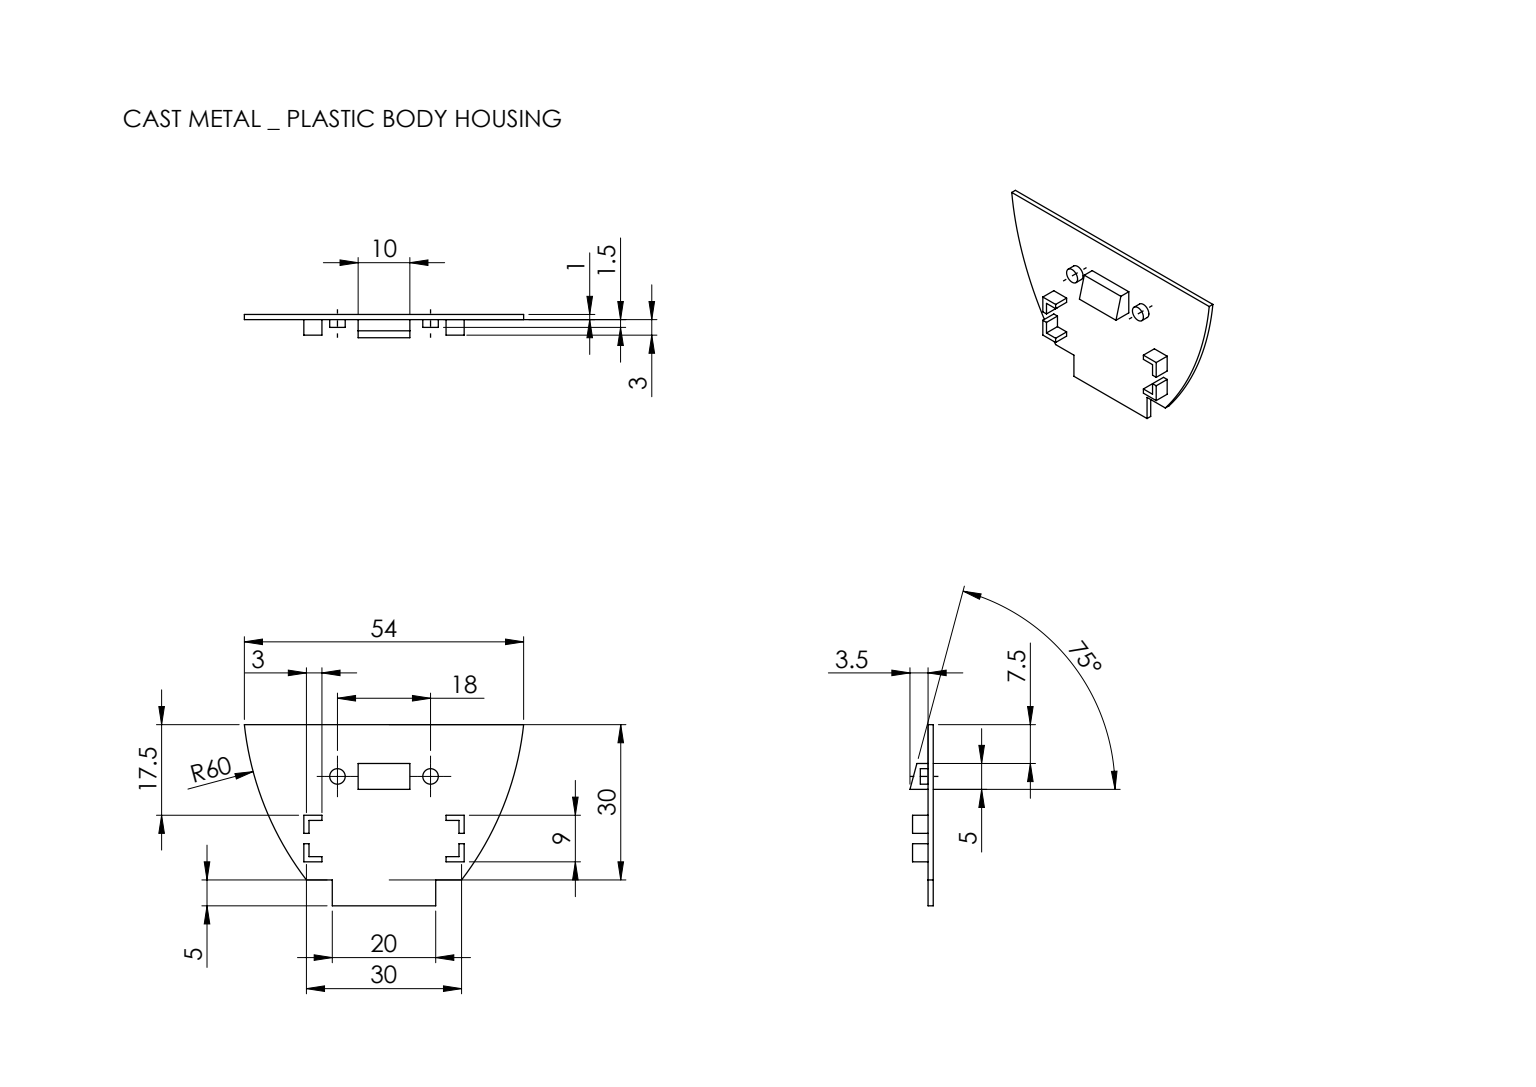
ISO-10303-21;
HEADER;
FILE_DESCRIPTION (('STEP AP214'),
    '1' );
FILE_NAME ('Cast Metal _ Plastic Body Housing.step',
    '2026-10-04T16:38:04',
    ( '' ),
    ( '' ),
    'SwSTEP 2.0',
    'SolidWorks 2026',
    '' );
FILE_SCHEMA (( 'AUTOMOTIVE_DESIGN' ));
ENDSEC;

DATA;
#46=DIRECTION ( 'NONE',  ( 1.000000000000000000, -6.938893903907222067E-15, 0.000000000000000000 ) ) ;
#48=EDGE_LOOP ( 'NONE', ( #6607, #18673, #6407, #16806 ) ) ;
#59=LINE ( 'NONE', #8216, #18452 ) ;
#71=ORIENTED_EDGE ( 'NONE', *, *, #17925, .T. ) ;
#150=EDGE_CURVE ( 'NONE', #20096, #3927, #16331, .T. ) ;
#155=EDGE_CURVE ( 'NONE', #9432, #10023, #14985, .T. ) ;
#189=ORIENTED_EDGE ( 'NONE', *, *, #9219, .F. ) ;
#198=EDGE_LOOP ( 'NONE', ( #19605, #1454, #13205, #13918 ) ) ;
#200=VERTEX_POINT ( 'NONE', #10184 ) ;
#212=DIRECTION ( 'NONE',  ( -1.000000000000000000, -6.938893903907222067E-15, 0.000000000000000000 ) ) ;
#216=ORIENTED_EDGE ( 'NONE', *, *, #5288, .T. ) ;
#237=CARTESIAN_POINT ( 'NONE',  ( 11.99999999999999822, -25.50000000000000355, 4.000000000000000000 ) ) ;
#244=ORIENTED_EDGE ( 'NONE', *, *, #20430, .T. ) ;
#247=LINE ( 'NONE', #19711, #19278 ) ;
#253=DIRECTION ( 'NONE',  ( 0.000000000000000000, 0.000000000000000000, -1.000000000000000000 ) ) ;
#254=EDGE_CURVE ( 'NONE', #12726, #11061, #10084, .T. ) ;
#255=CARTESIAN_POINT ( 'NONE',  ( -15.49999999999998046, -26.49999999999999645, 4.000000000000000000 ) ) ;
#297=VECTOR ( 'NONE', #5292, 1000.000000000000000 ) ;
#329=ORIENTED_EDGE ( 'NONE', *, *, #3787, .F. ) ;
#382=VERTEX_POINT ( 'NONE', #11949 ) ;
#383=ADVANCED_FACE ( 'NONE', ( #12259 ), #18550, .T. ) ;
#386=CARTESIAN_POINT ( 'NONE',  ( -14.99999999999998046, -26.49999999999999645, 4.000000000000000000 ) ) ;
#387=VECTOR ( 'NONE', #11320, 1000.000000000000000 ) ;
#398=AXIS2_PLACEMENT_3D ( 'NONE', #19475, #19368, #6705 ) ;
#408=ORIENTED_EDGE ( 'NONE', *, *, #19426, .T. ) ;
#437=DIRECTION ( 'NONE',  ( 1.000000000000000000, 5.204170427930411817E-15, -0.000000000000000000 ) ) ;
#452=VECTOR ( 'NONE', #1980, 1000.000000000000000 ) ;
#459=ADVANCED_FACE ( 'NONE', ( #3832 ), #17953, .T. ) ;
#462=DIRECTION ( 'NONE',  ( 1.000000000000000000, 0.000000000000000000, -0.000000000000000000 ) ) ;
#486=CARTESIAN_POINT ( 'NONE',  ( 15.00000000000001776, -26.49999999999999645, 1.000000000000000000 ) ) ;
#491=PLANE ( 'NONE',  #4290 ) ;
#498=ORIENTED_EDGE ( 'NONE', *, *, #11572, .F. ) ;
#514=VECTOR ( 'NONE', #18897, 1000.000000000000000 ) ;
#520=EDGE_CURVE ( 'NONE', #9432, #6659, #2464, .T. ) ;
#522=PLANE ( 'NONE',  #398 ) ;
#523=VECTOR ( 'NONE', #704, 1000.000000000000000 ) ;
#526=ORIENTED_EDGE ( 'NONE', *, *, #18607, .T. ) ;
#530=ADVANCED_FACE ( 'NONE', ( #697 ), #13548, .T. ) ;
#533=DIRECTION ( 'NONE',  ( 0.000000000000000000, 0.000000000000000000, 1.000000000000000000 ) ) ;
#535=FACE_OUTER_BOUND ( 'NONE', #13184, .T. ) ;
#551=VERTEX_POINT ( 'NONE', #2158 ) ;
#568=CARTESIAN_POINT ( 'NONE',  ( 15.50000000000000178, -20.99999999999999645, 4.000000000000000000 ) ) ;
#579=ORIENTED_EDGE ( 'NONE', *, *, #13507, .T. ) ;
#581=CARTESIAN_POINT ( 'NONE',  ( 15.50000000000000178, -23.00000000000000711, 1.000000000000000000 ) ) ;
#585=EDGE_LOOP ( 'NONE', ( #6013, #20660, #8946, #16986 ) ) ;
#599=EDGE_LOOP ( 'NONE', ( #16407, #1610, #13461, #14948 ) ) ;
#603=DIRECTION ( 'NONE',  ( 5.204170427930411817E-15, -1.000000000000000000, 0.000000000000000000 ) ) ;
#628=VECTOR ( 'NONE', #3098, 1000.000000000000000 ) ;
#642=VECTOR ( 'NONE', #3133, 1000.000000000000000 ) ;
#668=VECTOR ( 'NONE', #922, 1000.000000000000000 ) ;
#688=EDGE_LOOP ( 'NONE', ( #8301, #4160, #16182, #17775 ) ) ;
#697=FACE_OUTER_BOUND ( 'NONE', #48, .T. ) ;
#704=DIRECTION ( 'NONE',  ( -0.000000000000000000, -0.000000000000000000, -1.000000000000000000 ) ) ;
#722=CARTESIAN_POINT ( 'NONE',  ( 4.000000000000000000, -12.50000000000000000, 1.000000000000000000 ) ) ;
#745=AXIS2_PLACEMENT_3D ( 'NONE', #893, #13543, #3828 ) ;
#754=PRESENTATION_STYLE_ASSIGNMENT (( #11425 ) ) ;
#757=VECTOR ( 'NONE', #16963, 1000.000000000000000 ) ;
#787=ORIENTED_EDGE ( 'NONE', *, *, #12469, .F. ) ;
#794=LINE ( 'NONE', #11664, #1088 ) ;
#817=EDGE_LOOP ( 'NONE', ( #11943, #5676, #6063, #12462 ) ) ;
#831=ADVANCED_FACE ( 'NONE', ( #10843 ), #17206, .F. ) ;
#844=FILL_AREA_STYLE ('',( #8584 ) ) ;
#846=LINE ( 'NONE', #4289, #16135 ) ;
#849=CARTESIAN_POINT ( 'NONE',  ( -9.000000000000000000, -9.999999999999992895, 2.500000000000000000 ) ) ;
#868=VERTEX_POINT ( 'NONE', #2989 ) ;
#872=CARTESIAN_POINT ( 'NONE',  ( -27.00000000000000000, 0.000000000000000000, 1.000000000000000000 ) ) ;
#877=CARTESIAN_POINT ( 'NONE',  ( -12.00000000000000000, -25.49999999999998934, 4.000000000000000000 ) ) ;
#881=ORIENTED_EDGE ( 'NONE', *, *, #13059, .T. ) ;
#890=ORIENTED_EDGE ( 'NONE', *, *, #18715, .T. ) ;
#893=CARTESIAN_POINT ( 'NONE',  ( 32.65117217603048516, 6.460468870412194420, 0.000000000000000000 ) ) ;
#902=LINE ( 'NONE', #13241, #9957 ) ;
#911=VERTEX_POINT ( 'NONE', #11044 ) ;
#917=ORIENTED_EDGE ( 'NONE', *, *, #11391, .F. ) ;
#922=DIRECTION ( 'NONE',  ( -0.000000000000000000, -0.000000000000000000, -1.000000000000000000 ) ) ;
#967=FACE_OUTER_BOUND ( 'NONE', #17994, .T. ) ;
#990=AXIS2_PLACEMENT_3D ( 'NONE', #20222, #5883, #4722 ) ;
#1027=ORIENTED_EDGE ( 'NONE', *, *, #17853, .T. ) ;
#1035=PLANE ( 'NONE',  #7985 ) ;
#1036=FACE_OUTER_BOUND ( 'NONE', #17096, .T. ) ;
#1044=ORIENTED_EDGE ( 'NONE', *, *, #9355, .F. ) ;
#1057=ORIENTED_EDGE ( 'NONE', *, *, #3262, .T. ) ;
#1088=VECTOR ( 'NONE', #11873, 1000.000000000000000 ) ;
#1110=EDGE_CURVE ( 'NONE', #4929, #14114, #16258, .T. ) ;
#1124=PLANE ( 'NONE',  #12366 ) ;
#1151=CARTESIAN_POINT ( 'NONE',  ( -9.999999999999998224, -30.00000000000000355, 1.000000000000000000 ) ) ;
#1155=ORIENTED_EDGE ( 'NONE', *, *, #14762, .T. ) ;
#1195=EDGE_CURVE ( 'NONE', #18185, #20045, #9975, .T. ) ;
#1199=LINE ( 'NONE', #4441, #1374 ) ;
#1219=DIRECTION ( 'NONE',  ( -1.000000000000000000, 2.312964634635752916E-15, 0.000000000000000000 ) ) ;
#1231=VERTEX_POINT ( 'NONE', #2334 ) ;
#1244=CARTESIAN_POINT ( 'NONE',  ( 5.000000000000000000, -12.50000000000000000, 4.500000000000000888 ) ) ;
#1245=AXIS2_PLACEMENT_3D ( 'NONE', #6195, #6294, #8185 ) ;
#1255=DIRECTION ( 'NONE',  ( -3.469446951953611033E-15, -1.000000000000000000, 0.000000000000000000 ) ) ;
#1266=FACE_OUTER_BOUND ( 'NONE', #2611, .T. ) ;
#1276=ORIENTED_EDGE ( 'NONE', *, *, #16635, .F. ) ;
#1282=UNCERTAINTY_MEASURE_WITH_UNIT (LENGTH_MEASURE( 1.000000000000000082E-05 ), #8702, 'distance_accuracy_value', 'NONE');
#1284=DIRECTION ( 'NONE',  ( 3.469446951953611033E-15, 1.000000000000000000, 0.000000000000000000 ) ) ;
#1358=VECTOR ( 'NONE', #18316, 1000.000000000000000 ) ;
#1367=CARTESIAN_POINT ( 'NONE',  ( 15.00000000000001421, -29.99999999999998579, 0.000000000000000000 ) ) ;
#1374=VECTOR ( 'NONE', #12173, 1000.000000000000000 ) ;
#1375=VECTOR ( 'NONE', #5558, 1000.000000000000000 ) ;
#1408=EDGE_LOOP ( 'NONE', ( #15317, #16815, #12977, #18861, #4503, #15029 ) ) ;
#1412=DIRECTION ( 'NONE',  ( -6.938893903907222067E-15, -1.000000000000000000, 0.000000000000000000 ) ) ;
#1414=ORIENTED_EDGE ( 'NONE', *, *, #6972, .T. ) ;
#1424=CARTESIAN_POINT ( 'NONE',  ( -27.00000000000000000, 0.000000000000000000, 0.000000000000000000 ) ) ;
#1432=VECTOR ( 'NONE', #9969, 1000.000000000000000 ) ;
#1434=VERTEX_POINT ( 'NONE', #18655 ) ;
#1435=EDGE_CURVE ( 'NONE', #7660, #4902, #17180, .T. ) ;
#1454=ORIENTED_EDGE ( 'NONE', *, *, #17925, .F. ) ;
#1460=FACE_OUTER_BOUND ( 'NONE', #585, .T. ) ;
#1482=ORIENTED_EDGE ( 'NONE', *, *, #16635, .T. ) ;
#1489=CARTESIAN_POINT ( 'NONE',  ( -11.99999999999999467, -17.50000000000000000, 1.000000000000000000 ) ) ;
#1516=FACE_BOUND ( 'NONE', #16320, .T. ) ;
#1549=ORIENTED_EDGE ( 'NONE', *, *, #1825, .F. ) ;
#1557=ORIENTED_EDGE ( 'NONE', *, *, #15424, .F. ) ;
#1562=LINE ( 'NONE', #3235, #13129 ) ;
#1565=CARTESIAN_POINT ( 'NONE',  ( 4.000000000000000000, 0.000000000000000000, 0.000000000000000000 ) ) ;
#1571=PLANE ( 'NONE',  #11672 ) ;
#1594=LINE ( 'NONE', #7781, #15066 ) ;
#1601=VECTOR ( 'NONE', #13561, 1000.000000000000000 ) ;
#1604=ORIENTED_EDGE ( 'NONE', *, *, #18607, .F. ) ;
#1607=PLANE ( 'NONE',  #6334 ) ;
#1610=ORIENTED_EDGE ( 'NONE', *, *, #11754, .F. ) ;
#1620=DIRECTION ( 'NONE',  ( -1.000000000000000000, -3.469446951953611033E-15, 0.000000000000000000 ) ) ;
#1632=VECTOR ( 'NONE', #7369, 1000.000000000000000 ) ;
#1642=CARTESIAN_POINT ( 'NONE',  ( 10.00000000000000533, -30.00000000000000355, 0.000000000000000000 ) ) ;
#1647=LINE ( 'NONE', #12619, #3950 ) ;
#1695=ORIENTED_EDGE ( 'NONE', *, *, #9410, .F. ) ;
#1776=DIRECTION ( 'NONE',  ( -1.000000000000000000, 0.000000000000000000, 0.000000000000000000 ) ) ;
#1777=DIRECTION ( 'NONE',  ( 0.000000000000000000, -0.9659258262890672020, 0.2588190451025245142 ) ) ;
#1793=CARTESIAN_POINT ( 'NONE',  ( 0.000000000000000000, 0.000000000000000000, 0.000000000000000000 ) ) ;
#1799=PLANE ( 'NONE',  #15935 ) ;
#1820=ORIENTED_EDGE ( 'NONE', *, *, #15526, .F. ) ;
#1825=EDGE_CURVE ( 'NONE', #8456, #2576, #5382, .T. ) ;
#1828=CARTESIAN_POINT ( 'NONE',  ( 12.00000000000000178, -26.50000000000000355, 4.000000000000000000 ) ) ;
#1832=CARTESIAN_POINT ( 'NONE',  ( 15.00000000000001421, -25.49999999999999645, 1.000000000000000000 ) ) ;
#1845=ORIENTED_EDGE ( 'NONE', *, *, #9443, .T. ) ;
#1846=DIRECTION ( 'NONE',  ( 0.000000000000000000, -0.9659258262890672020, 0.2588190451025246253 ) ) ;
#1866=VERTEX_POINT ( 'NONE', #5666 ) ;
#1869=EDGE_LOOP ( 'NONE', ( #11250, #11872, #14832, #4061 ) ) ;
#1886=EDGE_CURVE ( 'NONE', #200, #2500, #20000, .T. ) ;
#1893=ORIENTED_EDGE ( 'NONE', *, *, #3662, .F. ) ;
#1900=LINE ( 'NONE', #11214, #20633 ) ;
#1901=DIRECTION ( 'NONE',  ( 0.000000000000000000, 0.000000000000000000, 1.000000000000000000 ) ) ;
#1924=CARTESIAN_POINT ( 'NONE',  ( -15.49999999999999822, -20.99999999999999645, 4.000000000000000000 ) ) ;
#1942=VERTEX_POINT ( 'NONE', #10685 ) ;
#1947=DIRECTION ( 'NONE',  ( 1.000000000000000000, 0.000000000000000000, 0.000000000000000000 ) ) ;
#1951=ORIENTED_EDGE ( 'NONE', *, *, #5701, .T. ) ;
#1953=DIRECTION ( 'NONE',  ( 0.000000000000000000, 0.000000000000000000, 1.000000000000000000 ) ) ;
#1978=CARTESIAN_POINT ( 'NONE',  ( -5.000000000000000000, -7.500000000000000000, 3.160254037844365094 ) ) ;
#1980=DIRECTION ( 'NONE',  ( 0.000000000000000000, 0.000000000000000000, -1.000000000000000000 ) ) ;
#1989=AXIS2_PLACEMENT_3D ( 'NONE', #16860, #18234, #9127 ) ;
#1990=EDGE_CURVE ( 'NONE', #13564, #6014, #16746, .T. ) ;
#1995=EDGE_LOOP ( 'NONE', ( #14834, #2151, #15596, #189, #1557, #14199, #4129, #1695 ) ) ;
#2006=PRODUCT_DEFINITION_SHAPE ( 'NONE', 'NONE',  #20327 ) ;
#2030=DIRECTION ( 'NONE',  ( 4.625929269271477434E-15, 1.000000000000000000, 0.000000000000000000 ) ) ;
#2033=CARTESIAN_POINT ( 'NONE',  ( -11.99999999999999467, -17.50000000000000000, 1.000000000000000000 ) ) ;
#2056=LINE ( 'NONE', #2458, #2757 ) ;
#2100=ORIENTED_EDGE ( 'NONE', *, *, #7749, .T. ) ;
#2104=DIRECTION ( 'NONE',  ( 0.000000000000000000, -0.9659258262890672020, 0.2588190451025245142 ) ) ;
#2108=ADVANCED_FACE ( 'NONE', ( #17469 ), #1571, .F. ) ;
#2121=VECTOR ( 'NONE', #12009, 1000.000000000000000 ) ;
#2150=ORIENTED_EDGE ( 'NONE', *, *, #4677, .T. ) ;
#2151=ORIENTED_EDGE ( 'NONE', *, *, #18217, .T. ) ;
#2158=CARTESIAN_POINT ( 'NONE',  ( 4.000000000000000000, -12.50000000000000000, 3.464723819589916154 ) ) ;
#2160=DIRECTION ( 'NONE',  ( -1.000000000000000000, -3.469446951953611033E-15, 0.000000000000000000 ) ) ;
#2167=ORIENTED_EDGE ( 'NONE', *, *, #14644, .T. ) ;
#2195=CARTESIAN_POINT ( 'NONE',  ( 12.00000000000000178, -18.50000000000000355, 1.000000000000000000 ) ) ;
#2200=( LENGTH_UNIT ( ) NAMED_UNIT ( * ) SI_UNIT ( .MILLI., .METRE. ) );
#2202=CARTESIAN_POINT ( 'NONE',  ( -14.49999999999999645, -22.99999999999998579, 4.000000000000000000 ) ) ;
#2228=DIRECTION ( 'NONE',  ( 0.000000000000000000, -1.000000000000000000, 0.000000000000000000 ) ) ;
#2235=LINE ( 'NONE', #6754, #14984 ) ;
#2238=ORIENTED_EDGE ( 'NONE', *, *, #3662, .T. ) ;
#2310=AXIS2_PLACEMENT_3D ( 'NONE', #2824, #11084, #17041 ) ;
#2334=CARTESIAN_POINT ( 'NONE',  ( 5.000000000000000000, -7.500000000000000000, 3.160254037844365094 ) ) ;
#2337=DIRECTION ( 'NONE',  ( -1.000000000000000000, 6.938893903907222067E-15, 0.000000000000000000 ) ) ;
#2353=ORIENTED_EDGE ( 'NONE', *, *, #254, .F. ) ;
#2355=ORIENTED_EDGE ( 'NONE', *, *, #20532, .T. ) ;
#2359=LINE ( 'NONE', #5401, #7994 ) ;
#2378=ORIENTED_EDGE ( 'NONE', *, *, #19426, .F. ) ;
#2383=ORIENTED_EDGE ( 'NONE', *, *, #1435, .T. ) ;
#2390=CARTESIAN_POINT ( 'NONE',  ( 10.49999999999999467, -9.999999999999991118, 2.500000000000000000 ) ) ;
#2455=CARTESIAN_POINT ( 'NONE',  ( 15.50000000000002132, -26.49999999999999645, 1.000000000000000000 ) ) ;
#2458=CARTESIAN_POINT ( 'NONE',  ( 12.00000000000000178, -26.50000000000000355, 1.000000000000000000 ) ) ;
#2464=LINE ( 'NONE', #4042, #297 ) ;
#2467=EDGE_CURVE ( 'NONE', #19883, #3190, #5533, .T. ) ;
#2469=CARTESIAN_POINT ( 'NONE',  ( 5.000000000000000000, -12.50000000000000000, 1.000000000000000000 ) ) ;
#2474=ORIENTED_EDGE ( 'NONE', *, *, #4002, .T. ) ;
#2477=VERTEX_POINT ( 'NONE', #18608 ) ;
#2483=VERTEX_POINT ( 'NONE', #12219 ) ;
#2500=VERTEX_POINT ( 'NONE', #17028 ) ;
#2501=EDGE_CURVE ( 'NONE', #6659, #14414, #4070, .T. ) ;
#2506=( NAMED_UNIT ( * ) SI_UNIT ( $, .STERADIAN. ) SOLID_ANGLE_UNIT ( ) );
#2566=DIRECTION ( 'NONE',  ( 0.000000000000000000, 0.000000000000000000, 1.000000000000000000 ) ) ;
#2576=VERTEX_POINT ( 'NONE', #15251 ) ;
#2600=ORIENTED_EDGE ( 'NONE', *, *, #7451, .T. ) ;
#2611=EDGE_LOOP ( 'NONE', ( #2600, #7746, #1044, #15474 ) ) ;
#2614=ORIENTED_EDGE ( 'NONE', *, *, #1886, .T. ) ;
#2617=LINE ( 'NONE', #15380, #14540 ) ;
#2664=EDGE_LOOP ( 'NONE', ( #6791, #7977 ) ) ;
#2671=VECTOR ( 'NONE', #17590, 1000.000000000000000 ) ;
#2714=ORIENTED_EDGE ( 'NONE', *, *, #11572, .T. ) ;
#2719=LINE ( 'NONE', #10978, #19024 ) ;
#2752=CARTESIAN_POINT ( 'NONE',  ( 10.00000000000000533, -30.00000000000000355, 1.000000000000000000 ) ) ;
#2757=VECTOR ( 'NONE', #5396, 1000.000000000000000 ) ;
#2761=DIRECTION ( 'NONE',  ( -1.000000000000000000, 0.000000000000000000, 0.000000000000000000 ) ) ;
#2767=CARTESIAN_POINT ( 'NONE',  ( -7.500000000000000888, -9.999999999999992895, 1.000000000000000000 ) ) ;
#2777=EDGE_CURVE ( 'NONE', #18339, #6572, #8684, .T. ) ;
#2810=DIRECTION ( 'NONE',  ( 0.000000000000000000, 0.000000000000000000, -1.000000000000000000 ) ) ;
#2813=DIRECTION ( 'NONE',  ( 1.000000000000000000, 0.000000000000000000, 0.000000000000000000 ) ) ;
#2824=CARTESIAN_POINT ( 'NONE',  ( -12.00000000000000000, -25.49999999999998934, 4.000000000000000000 ) ) ;
#2828=PRODUCT ( 'Cast Metal _ Plastic Body Housing', 'Cast Metal _ Plastic Body Housing', '', ( #13255 ) ) ;
#2832=EDGE_LOOP ( 'NONE', ( #2167, #408, #579, #12559, #3746, #13946, #2355, #2238 ) ) ;
#2878=EDGE_CURVE ( 'NONE', #17965, #11811, #14580, .T. ) ;
#2889=FACE_OUTER_BOUND ( 'NONE', #9746, .T. ) ;
#2906=ORIENTED_EDGE ( 'NONE', *, *, #11391, .T. ) ;
#2909=VECTOR ( 'NONE', #5961, 1000.000000000000000 ) ;
#2911=CARTESIAN_POINT ( 'NONE',  ( 27.00000000000000000, 0.000000000000000000, 0.000000000000000000 ) ) ;
#2923=CARTESIAN_POINT ( 'NONE',  ( -14.99999999999998401, -25.49999999999999645, 4.000000000000000000 ) ) ;
#2956=AXIS2_PLACEMENT_3D ( 'NONE', #8491, #18002, #5454 ) ;
#2974=CARTESIAN_POINT ( 'NONE',  ( -11.99999999999999645, -26.49999999999998934, 4.000000000000000000 ) ) ;
#2976=ORIENTED_EDGE ( 'NONE', *, *, #20430, .F. ) ;
#2986=DIRECTION ( 'NONE',  ( -1.000000000000000000, -0.000000000000000000, -0.000000000000000000 ) ) ;
#2989=CARTESIAN_POINT ( 'NONE',  ( -12.00000000000000000, -25.49999999999998934, 4.000000000000000000 ) ) ;
#2999=EDGE_CURVE ( 'NONE', #868, #11896, #3164, .T. ) ;
#3007=ORIENTED_EDGE ( 'NONE', *, *, #5387, .F. ) ;
#3019=CARTESIAN_POINT ( 'NONE',  ( 14.50000000000000000, -23.00000000000001421, 1.000000000000000000 ) ) ;
#3020=CARTESIAN_POINT ( 'NONE',  ( 14.50000000000000000, -20.99999999999998934, 4.000000000000000000 ) ) ;
#3046=VECTOR ( 'NONE', #4131, 1000.000000000000000 ) ;
#3067=CARTESIAN_POINT ( 'NONE',  ( 12.00000000000000178, -26.50000000000000355, 4.000000000000000000 ) ) ;
#3089=VECTOR ( 'NONE', #8023, 1000.000000000000000 ) ;
#3093=CARTESIAN_POINT ( 'NONE',  ( -15.49999999999999822, -22.99999999999999289, 4.000000000000000000 ) ) ;
#3098=DIRECTION ( 'NONE',  ( -1.000000000000000000, -0.000000000000000000, -0.000000000000000000 ) ) ;
#3111=CARTESIAN_POINT ( 'NONE',  ( 15.50000000000000178, -20.99999999999999645, 4.000000000000000000 ) ) ;
#3113=CARTESIAN_POINT ( 'NONE',  ( 15.50000000000000178, -23.00000000000000711, 4.000000000000000000 ) ) ;
#3118=AXIS2_PLACEMENT_3D ( 'NONE', #17355, #11282, #17665 ) ;
#3122=CARTESIAN_POINT ( 'NONE',  ( -4.000000000000000000, -12.50000000000000000, 3.464723819589916154 ) ) ;
#3133=DIRECTION ( 'NONE',  ( 1.000000000000000000, 6.938893903907232322E-16, 0.000000000000000000 ) ) ;
#3144=CARTESIAN_POINT ( 'NONE',  ( -4.000000000000000000, -8.500000000000000000, 2.392927049865408495 ) ) ;
#3164=LINE ( 'NONE', #6409, #13702 ) ;
#3183=CARTESIAN_POINT ( 'NONE',  ( -10.49999999999999822, -9.999999999999992895, 1.000000000000000000 ) ) ;
#3185=ORIENTED_EDGE ( 'NONE', *, *, #1435, .F. ) ;
#3188=EDGE_CURVE ( 'NONE', #16474, #4026, #16739, .T. ) ;
#3190=VERTEX_POINT ( 'NONE', #13496 ) ;
#3191=LINE ( 'NONE', #17904, #16020 ) ;
#3196=CARTESIAN_POINT ( 'NONE',  ( 10.49999999999999645, -9.999999999999991118, 1.000000000000000000 ) ) ;
#3235=CARTESIAN_POINT ( 'NONE',  ( 12.00000000000000178, -18.50000000000000355, 1.000000000000000000 ) ) ;
#3236=ORIENTED_EDGE ( 'NONE', *, *, #13283, .F. ) ;
#3262=EDGE_CURVE ( 'NONE', #12726, #19461, #13391, .T. ) ;
#3307=VECTOR ( 'NONE', #19013, 1000.000000000000000 ) ;
#3311=DIRECTION ( 'NONE',  ( 0.000000000000000000, 0.000000000000000000, -1.000000000000000000 ) ) ;
#3363=EDGE_LOOP ( 'NONE', ( #17972, #9302, #11307, #5959 ) ) ;
#3364=DIRECTION ( 'NONE',  ( 0.000000000000000000, -0.2588190451025247363, -0.9659258262890673130 ) ) ;
#3379=ORIENTED_EDGE ( 'NONE', *, *, #14251, .F. ) ;
#3399=FACE_OUTER_BOUND ( 'NONE', #19377, .T. ) ;
#3407=EDGE_CURVE ( 'NONE', #19990, #7441, #12504, .T. ) ;
#3412=CARTESIAN_POINT ( 'NONE',  ( -10.49999999999999822, -9.999999999999992895, 2.500000000000000000 ) ) ;
#3421=VECTOR ( 'NONE', #18309, 1000.000000000000000 ) ;
#3423=ADVANCED_FACE ( 'NONE', ( #2889 ), #1124, .F. ) ;
#3424=PLANE ( 'NONE',  #8675 ) ;
#3449=ADVANCED_FACE ( 'NONE', ( #18901 ), #4559, .T. ) ;
#3465=EDGE_LOOP ( 'NONE', ( #16160, #5425, #10306, #917, #71, #16273, #4474, #10670 ) ) ;
#3471=FACE_BOUND ( 'NONE', #1995, .T. ) ;
#3505=ORIENTED_EDGE ( 'NONE', *, *, #1195, .T. ) ;
#3509=ORIENTED_EDGE ( 'NONE', *, *, #5846, .T. ) ;
#3539=CARTESIAN_POINT ( 'NONE',  ( 7.500000000000002665, -9.999999999999991118, 2.500000000000000000 ) ) ;
#3547=CARTESIAN_POINT ( 'NONE',  ( 14.50000000000000000, -23.00000000000001421, 4.000000000000000000 ) ) ;
#3548=DIRECTION ( 'NONE',  ( 1.000000000000000000, 2.312964634635756072E-15, 0.000000000000000000 ) ) ;
#3555=FACE_OUTER_BOUND ( 'NONE', #4637, .T. ) ;
#3566=CARTESIAN_POINT ( 'NONE',  ( -14.49999999999998401, -25.49999999999999645, 1.000000000000000000 ) ) ;
#3575=CARTESIAN_POINT ( 'NONE',  ( 27.00000000000000000, 0.000000000000000000, 1.000000000000000000 ) ) ;
#3599=CIRCLE ( 'NONE', #16625, 1.499999999999996225 ) ;
#3611=ORIENTED_EDGE ( 'NONE', *, *, #19595, .F. ) ;
#3644=ORIENTED_EDGE ( 'NONE', *, *, #9219, .T. ) ;
#3662=EDGE_CURVE ( 'NONE', #20379, #13564, #9476, .T. ) ;
#3728=EDGE_LOOP ( 'NONE', ( #17200, #16705, #11798, #9456 ) ) ;
#3733=CARTESIAN_POINT ( 'NONE',  ( 12.00000000000000178, -18.50000000000000355, 4.000000000000000000 ) ) ;
#3746=ORIENTED_EDGE ( 'NONE', *, *, #6940, .T. ) ;
#3776=CARTESIAN_POINT ( 'NONE',  ( 5.000000000000000000, -12.50000000000000000, 1.000000000000000000 ) ) ;
#3779=DIRECTION ( 'NONE',  ( 1.000000000000000000, 2.312964634635756072E-15, 0.000000000000000000 ) ) ;
#3787=EDGE_CURVE ( 'NONE', #17877, #19250, #1199, .T. ) ;
#3828=DIRECTION ( 'NONE',  ( 1.000000000000000000, 0.000000000000000000, 0.000000000000000000 ) ) ;
#3832=FACE_OUTER_BOUND ( 'NONE', #3363, .T. ) ;
#3836=DIRECTION ( 'NONE',  ( -0.000000000000000000, -0.000000000000000000, -1.000000000000000000 ) ) ;
#3874=PRESENTATION_STYLE_ASSIGNMENT (( #16839 ) ) ;
#3894=ORIENTED_EDGE ( 'NONE', *, *, #3407, .F. ) ;
#3922=VERTEX_POINT ( 'NONE', #17089 ) ;
#3923=ORIENTED_EDGE ( 'NONE', *, *, #8620, .F. ) ;
#3927=VERTEX_POINT ( 'NONE', #2767 ) ;
#3941=VERTEX_POINT ( 'NONE', #17396 ) ;
#3950=VECTOR ( 'NONE', #17641, 1000.000000000000000 ) ;
#3955=FACE_OUTER_BOUND ( 'NONE', #9914, .T. ) ;
#3963=ORIENTED_EDGE ( 'NONE', *, *, #150, .T. ) ;
#3972=ORIENTED_EDGE ( 'NONE', *, *, #6354, .F. ) ;
#4002=EDGE_CURVE ( 'NONE', #4902, #3922, #16147, .T. ) ;
#4008=VECTOR ( 'NONE', #5945, 1000.000000000000000 ) ;
#4010=DIRECTION ( 'NONE',  ( -1.000000000000000000, 0.000000000000000000, 0.000000000000000000 ) ) ;
#4011=CARTESIAN_POINT ( 'NONE',  ( 5.000000000000000000, -12.50000000000000000, 1.000000000000000000 ) ) ;
#4014=LINE ( 'NONE', #877, #5736 ) ;
#4026=VERTEX_POINT ( 'NONE', #6625 ) ;
#4028=LINE ( 'NONE', #9051, #13052 ) ;
#4032=ORIENTED_EDGE ( 'NONE', *, *, #1886, .F. ) ;
#4042=CARTESIAN_POINT ( 'NONE',  ( -15.49999999999999822, -20.99999999999999645, 4.000000000000000000 ) ) ;
#4057=AXIS2_PLACEMENT_3D ( 'NONE', #5691, #15608, #2761 ) ;
#4061=ORIENTED_EDGE ( 'NONE', *, *, #18921, .T. ) ;
#4068=FACE_OUTER_BOUND ( 'NONE', #8866, .T. ) ;
#4070=LINE ( 'NONE', #12010, #4008 ) ;
#4084=( NAMED_UNIT ( * ) SI_UNIT ( $, .STERADIAN. ) SOLID_ANGLE_UNIT ( ) );
#4100=PLANE ( 'NONE',  #16718 ) ;
#4120=CYLINDRICAL_SURFACE ( 'NONE', #4057, 1.499999999999996891 ) ;
#4129=ORIENTED_EDGE ( 'NONE', *, *, #15235, .T. ) ;
#4131=DIRECTION ( 'NONE',  ( -0.000000000000000000, -0.000000000000000000, -1.000000000000000000 ) ) ;
#4134=LINE ( 'NONE', #5394, #11484 ) ;
#4144=CARTESIAN_POINT ( 'NONE',  ( -4.000000000000000000, -8.500000000000000000, 1.000000000000000000 ) ) ;
#4147=CARTESIAN_POINT ( 'NONE',  ( 0.000000000000000000, 0.000000000000000000, 4.000000000000000000 ) ) ;
#4160=ORIENTED_EDGE ( 'NONE', *, *, #520, .F. ) ;
#4185=LINE ( 'NONE', #15575, #2909 ) ;
#4189=CIRCLE ( 'NONE', #18271, 1.499999999999996225 ) ;
#4193=AXIS2_PLACEMENT_3D ( 'NONE', #1828, #1620, #12703 ) ;
#4196=CARTESIAN_POINT ( 'NONE',  ( 9.000000000000000000, -9.999999999999991118, 2.500000000000000000 ) ) ;
#4201=CARTESIAN_POINT ( 'NONE',  ( -15.49999999999999822, -22.99999999999999289, 4.000000000000000000 ) ) ;
#4214=CARTESIAN_POINT ( 'NONE',  ( -9.000000000000000000, -9.999999999999992895, 2.500000000000000000 ) ) ;
#4232=ORIENTED_EDGE ( 'NONE', *, *, #7719, .F. ) ;
#4234=CARTESIAN_POINT ( 'NONE',  ( 4.000000000000000000, -8.500000000000000000, 1.000000000000000000 ) ) ;
#4253=ADVANCED_FACE ( 'NONE', ( #18145 ), #16360, .T. ) ;
#4259=CARTESIAN_POINT ( 'NONE',  ( -11.99999999999999822, -18.50000000000000355, 1.000000000000000000 ) ) ;
#4281=DIRECTION ( 'NONE',  ( -3.469446951953619119E-16, -1.000000000000000000, 0.000000000000000000 ) ) ;
#4285=CARTESIAN_POINT ( 'NONE',  ( -15.49999999999998224, -17.49999999999999645, 1.000000000000000000 ) ) ;
#4289=CARTESIAN_POINT ( 'NONE',  ( 15.50000000000000178, -23.00000000000000711, 4.000000000000000000 ) ) ;
#4290=AXIS2_PLACEMENT_3D ( 'NONE', #3733, #2160, #13960 ) ;
#4299=AXIS2_PLACEMENT_3D ( 'NONE', #10111, #10211, #16578 ) ;
#4300=CARTESIAN_POINT ( 'NONE',  ( 14.50000000000000000, -20.99999999999998934, 4.000000000000000000 ) ) ;
#4313=ORIENTED_EDGE ( 'NONE', *, *, #16286, .F. ) ;
#4317=EDGE_CURVE ( 'NONE', #12726, #9432, #18246, .T. ) ;
#4340=ORIENTED_EDGE ( 'NONE', *, *, #7759, .F. ) ;
#4345=CARTESIAN_POINT ( 'NONE',  ( -9.999999999999996447, -34.99999999999999289, 0.000000000000000000 ) ) ;
#4351=CARTESIAN_POINT ( 'NONE',  ( 15.00000000000001421, -17.49999999999999645, 4.000000000000000000 ) ) ;
#4353=CARTESIAN_POINT ( 'NONE',  ( -14.99999999999998579, -18.49999999999999645, 4.000000000000000000 ) ) ;
#4356=LINE ( 'NONE', #18690, #15295 ) ;
#4378=FACE_OUTER_BOUND ( 'NONE', #11821, .T. ) ;
#4381=CARTESIAN_POINT ( 'NONE',  ( -9.999999999999996447, -34.99999999999999289, 1.000000000000000000 ) ) ;
#4394=PLANE ( 'NONE',  #2310 ) ;
#4399=ORIENTED_EDGE ( 'NONE', *, *, #19975, .T. ) ;
#4408=DIRECTION ( 'NONE',  ( 1.000000000000000000, 0.000000000000000000, 0.000000000000000000 ) ) ;
#4424=AXIS2_PLACEMENT_3D ( 'NONE', #18262, #15423, #8746 ) ;
#4426=ADVANCED_FACE ( 'NONE', ( #10400 ), #4120, .T. ) ;
#4441=CARTESIAN_POINT ( 'NONE',  ( 12.00000000000000178, -18.50000000000000355, 4.000000000000000000 ) ) ;
#4442=EDGE_CURVE ( 'NONE', #868, #5651, #4014, .T. ) ;
#4474=ORIENTED_EDGE ( 'NONE', *, *, #1110, .F. ) ;
#4484=DIRECTION ( 'NONE',  ( 0.000000000000000000, 0.000000000000000000, -1.000000000000000000 ) ) ;
#4492=VERTEX_POINT ( 'NONE', #17183 ) ;
#4500=ORIENTED_EDGE ( 'NONE', *, *, #1195, .F. ) ;
#4503=ORIENTED_EDGE ( 'NONE', *, *, #9517, .T. ) ;
#4522=DIRECTION ( 'NONE',  ( 3.469446951953619119E-16, 1.000000000000000000, -0.000000000000000000 ) ) ;
#4552=CARTESIAN_POINT ( 'NONE',  ( -27.00000000000000000, 0.000000000000000000, 0.000000000000000000 ) ) ;
#4554=DIRECTION ( 'NONE',  ( 1.000000000000000000, 2.312964634635731617E-15, 0.000000000000000000 ) ) ;
#4556=DIRECTION ( 'NONE',  ( 0.000000000000000000, 0.000000000000000000, 1.000000000000000000 ) ) ;
#4559=PLANE ( 'NONE',  #4694 ) ;
#4579=LINE ( 'NONE', #7521, #5635 ) ;
#4626=FACE_OUTER_BOUND ( 'NONE', #8654, .T. ) ;
#4632=ADVANCED_FACE ( 'NONE', ( #17492 ), #7974, .F. ) ;
#4637=EDGE_LOOP ( 'NONE', ( #14176, #5450, #16840, #20274 ) ) ;
#4642=VERTEX_POINT ( 'NONE', #12571 ) ;
#4647=CARTESIAN_POINT ( 'NONE',  ( -15.49999999999998224, -17.49999999999999645, 4.000000000000000000 ) ) ;
#4677=EDGE_CURVE ( 'NONE', #11061, #12047, #14236, .T. ) ;
#4694=AXIS2_PLACEMENT_3D ( 'NONE', #12294, #10628, #7703 ) ;
#4696=CARTESIAN_POINT ( 'NONE',  ( 10.00000000000000533, -30.00000000000000355, 1.000000000000000000 ) ) ;
#4698=DIRECTION ( 'NONE',  ( 0.000000000000000000, 0.000000000000000000, 1.000000000000000000 ) ) ;
#4722=DIRECTION ( 'NONE',  ( -1.000000000000000000, 0.000000000000000000, 0.000000000000000000 ) ) ;
#4750=EDGE_LOOP ( 'NONE', ( #8302, #6285, #8715, #4399 ) ) ;
#4754=EDGE_CURVE ( 'NONE', #382, #14114, #4940, .T. ) ;
#4760=DIRECTION ( 'NONE',  ( -1.000000000000000000, 2.312964634635752916E-15, 0.000000000000000000 ) ) ;
#4777=EDGE_CURVE ( 'NONE', #5036, #19990, #1594, .T. ) ;
#4788=LINE ( 'NONE', #10116, #6284 ) ;
#4802=ADVANCED_FACE ( 'NONE', ( #4626 ), #9546, .T. ) ;
#4808=DIRECTION ( 'NONE',  ( -3.469446951953611033E-15, 1.000000000000000000, 0.000000000000000000 ) ) ;
#4812=CARTESIAN_POINT ( 'NONE',  ( -9.999999999999998224, -30.00000000000000355, 1.000000000000000000 ) ) ;
#4871=VERTEX_POINT ( 'NONE', #11426 ) ;
#4875=EDGE_CURVE ( 'NONE', #20379, #10445, #11733, .T. ) ;
#4879=PLANE ( 'NONE',  #6767 ) ;
#4885=LINE ( 'NONE', #3122, #17981 ) ;
#4902=VERTEX_POINT ( 'NONE', #16633 ) ;
#4928=VERTEX_POINT ( 'NONE', #11527 ) ;
#4929=VERTEX_POINT ( 'NONE', #13291 ) ;
#4934=CARTESIAN_POINT ( 'NONE',  ( 4.000000000000000000, -12.50000000000000000, 1.000000000000000000 ) ) ;
#4940=LINE ( 'NONE', #6521, #387 ) ;
#4957=CLOSED_SHELL ( 'NONE', ( #4426, #8724, #15599, #4802, #15798, #5412, #4632, #19562, #12719, #530, #8440, #6806, #383, #10255, #459, #10301, #16890, #7051, #17076, #9542, #20019, #8582, #10441, #831, #16791, #5261, #5051, #13923, #2108, #16643, #20503, #17154, #11687, #16299, #4253, #19070, #3423, #6179, #19588, #19597, #7308, #12742, #12322, #7848, #9423, #7126, #8404, #3449, #6150, #16964, #16043, #8605, #8840 ) ) ;
#4969=AXIS2_PLACEMENT_3D ( 'NONE', #19636, #15222, #5607 ) ;
#4980=LINE ( 'NONE', #16076, #18086 ) ;
#4985=ORIENTED_EDGE ( 'NONE', *, *, #9443, .F. ) ;
#4994=CARTESIAN_POINT ( 'NONE',  ( -14.49999999999998579, -18.49999999999999645, 4.000000000000000000 ) ) ;
#5014=LINE ( 'NONE', #4812, #5121 ) ;
#5036=VERTEX_POINT ( 'NONE', #17163 ) ;
#5048=SURFACE_SIDE_STYLE ('',( #19390 ) ) ;
#5051=ADVANCED_FACE ( 'NONE', ( #15180 ), #20004, .T. ) ;
#5059=ORIENTED_EDGE ( 'NONE', *, *, #14111, .F. ) ;
#5077=DIRECTION ( 'NONE',  ( -1.000000000000000000, -2.312964634635730039E-15, 0.000000000000000000 ) ) ;
#5115=AXIS2_PLACEMENT_3D ( 'NONE', #8802, #8900, #15170 ) ;
#5121=VECTOR ( 'NONE', #14424, 1000.000000000000000 ) ;
#5129=CARTESIAN_POINT ( 'NONE',  ( 15.00000000000000355, -30.00000000000000000, 1.000000000000000000 ) ) ;
#5130=DIRECTION ( 'NONE',  ( 1.000000000000000000, 2.312964634635756072E-15, 0.000000000000000000 ) ) ;
#5140=ORIENTED_EDGE ( 'NONE', *, *, #2501, .T. ) ;
#5144=CARTESIAN_POINT ( 'NONE',  ( 10.00000000000000355, -34.99999999999999289, 0.000000000000000000 ) ) ;
#5165=DIRECTION ( 'NONE',  ( 1.000000000000000000, 0.000000000000000000, 0.000000000000000000 ) ) ;
#5183=AXIS2_PLACEMENT_3D ( 'NONE', #10261, #7338, #18120 ) ;
#5210=ORIENTED_EDGE ( 'NONE', *, *, #4777, .T. ) ;
#5218=CIRCLE ( 'NONE', #6894, 1.499999999999996225 ) ;
#5225=DIRECTION ( 'NONE',  ( -6.938893903907232322E-16, 1.000000000000000000, 0.000000000000000000 ) ) ;
#5227=AXIS2_PLACEMENT_3D ( 'NONE', #4353, #5823, #1219 ) ;
#5260=CARTESIAN_POINT ( 'NONE',  ( 32.65117217603048516, 6.460468870412194420, 0.000000000000000000 ) ) ;
#5261=ADVANCED_FACE ( 'NONE', ( #12965 ), #522, .T. ) ;
#5288=EDGE_CURVE ( 'NONE', #7441, #5651, #5442, .T. ) ;
#5292=DIRECTION ( 'NONE',  ( -0.000000000000000000, -0.000000000000000000, -1.000000000000000000 ) ) ;
#5294=CARTESIAN_POINT ( 'NONE',  ( -15.49999999999999822, -22.99999999999999289, 4.000000000000000000 ) ) ;
#5370=CARTESIAN_POINT ( 'NONE',  ( -14.99999999999998224, -17.49999999999999645, 1.000000000000000000 ) ) ;
#5371=DIRECTION ( 'NONE',  ( -0.000000000000000000, -0.000000000000000000, -1.000000000000000000 ) ) ;
#5374=DIRECTION ( 'NONE',  ( -1.000000000000000000, -0.000000000000000000, -0.000000000000000000 ) ) ;
#5378=AXIS2_PLACEMENT_3D ( 'NONE', #11020, #6419, #17389 ) ;
#5382=CIRCLE ( 'NONE', #8393, 1.499999999999996225 ) ;
#5387=EDGE_CURVE ( 'NONE', #19732, #14809, #15159, .T. ) ;
#5389=ORIENTED_EDGE ( 'NONE', *, *, #2777, .F. ) ;
#5394=CARTESIAN_POINT ( 'NONE',  ( -14.99999999999998579, -18.49999999999999645, 1.000000000000000000 ) ) ;
#5396=DIRECTION ( 'NONE',  ( -3.469446951953611033E-15, 1.000000000000000000, 0.000000000000000000 ) ) ;
#5401=CARTESIAN_POINT ( 'NONE',  ( -5.000000000000000000, -12.50000000000000000, 1.000000000000000000 ) ) ;
#5402=FACE_OUTER_BOUND ( 'NONE', #14924, .T. ) ;
#5412=ADVANCED_FACE ( 'NONE', ( #11911 ), #13892, .F. ) ;
#5417=ORIENTED_EDGE ( 'NONE', *, *, #5846, .F. ) ;
#5425=ORIENTED_EDGE ( 'NONE', *, *, #16145, .T. ) ;
#5431=LINE ( 'NONE', #19973, #7024 ) ;
#5442=LINE ( 'NONE', #13381, #12752 ) ;
#5447=ORIENTED_EDGE ( 'NONE', *, *, #1825, .T. ) ;
#5450=ORIENTED_EDGE ( 'NONE', *, *, #7749, .F. ) ;
#5454=DIRECTION ( 'NONE',  ( -5.204170427930446527E-15, 1.000000000000000000, 0.000000000000000000 ) ) ;
#5461=FILL_AREA_STYLE ('',( #12989 ) ) ;
#5471=PLANE ( 'NONE',  #1989 ) ;
#5496=ORIENTED_EDGE ( 'NONE', *, *, #16286, .T. ) ;
#5498=ORIENTED_EDGE ( 'NONE', *, *, #4875, .T. ) ;
#5533=LINE ( 'NONE', #4381, #14343 ) ;
#5558=DIRECTION ( 'NONE',  ( -0.000000000000000000, -0.000000000000000000, -1.000000000000000000 ) ) ;
#5597=LINE ( 'NONE', #20043, #3046 ) ;
#5607=DIRECTION ( 'NONE',  ( -1.000000000000000000, 0.000000000000000000, 0.000000000000000000 ) ) ;
#5627=EDGE_LOOP ( 'NONE', ( #4985, #8971, #15114, #498 ) ) ;
#5629=LINE ( 'NONE', #12005, #16653 ) ;
#5635=VECTOR ( 'NONE', #13885, 1000.000000000000000 ) ;
#5636=VECTOR ( 'NONE', #17223, 1000.000000000000000 ) ;
#5651=VERTEX_POINT ( 'NONE', #12433 ) ;
#5654=SURFACE_STYLE_FILL_AREA ( #844 ) ;
#5666=CARTESIAN_POINT ( 'NONE',  ( 5.000000000000000000, -12.50000000000000000, 4.500000000000000888 ) ) ;
#5676=ORIENTED_EDGE ( 'NONE', *, *, #10058, .F. ) ;
#5691=CARTESIAN_POINT ( 'NONE',  ( 9.000000000000000000, -9.999999999999991118, 2.500000000000000000 ) ) ;
#5701=EDGE_CURVE ( 'NONE', #20045, #4642, #20604, .T. ) ;
#5711=VERTEX_POINT ( 'NONE', #15876 ) ;
#5724=CARTESIAN_POINT ( 'NONE',  ( -5.000000000000000000, -7.500000000000000000, 3.160254037844365094 ) ) ;
#5736=VECTOR ( 'NONE', #20135, 1000.000000000000000 ) ;
#5748=VECTOR ( 'NONE', #6643, 1000.000000000000000 ) ;
#5776=AXIS2_PLACEMENT_3D ( 'NONE', #2202, #437, #19795 ) ;
#5787=CARTESIAN_POINT ( 'NONE',  ( -11.99999999999999467, -17.50000000000000000, 4.000000000000000000 ) ) ;
#5793=CARTESIAN_POINT ( 'NONE',  ( 15.00000000000001421, -25.49999999999999645, 4.000000000000000000 ) ) ;
#5805=EDGE_LOOP ( 'NONE', ( #12151, #15573, #2353, #1057 ) ) ;
#5818=LINE ( 'NONE', #9061, #14336 ) ;
#5823=DIRECTION ( 'NONE',  ( 2.312964634635752916E-15, 1.000000000000000000, -0.000000000000000000 ) ) ;
#5846=EDGE_CURVE ( 'NONE', #9650, #1231, #20262, .T. ) ;
#5849=PLANE ( 'NONE',  #7959 ) ;
#5864=LINE ( 'NONE', #16937, #13915 ) ;
#5869=DIRECTION ( 'NONE',  ( -0.000000000000000000, -0.000000000000000000, -1.000000000000000000 ) ) ;
#5875=DIRECTION ( 'NONE',  ( -4.625929269271486111E-15, -1.000000000000000000, 0.000000000000000000 ) ) ;
#5883=DIRECTION ( 'NONE',  ( 0.000000000000000000, 0.000000000000000000, 1.000000000000000000 ) ) ;
#5886=ORIENTED_EDGE ( 'NONE', *, *, #8574, .F. ) ;
#5895=CARTESIAN_POINT ( 'NONE',  ( -9.999999999999996447, -34.99999999999999289, 1.000000000000000000 ) ) ;
#5906=ORIENTED_EDGE ( 'NONE', *, *, #5288, .F. ) ;
#5921=CARTESIAN_POINT ( 'NONE',  ( 5.000000000000000000, -7.500000000000000000, 1.000000000000000000 ) ) ;
#5943=DIRECTION ( 'NONE',  ( -1.000000000000000000, 0.000000000000000000, 0.000000000000000000 ) ) ;
#5944=EDGE_CURVE ( 'NONE', #12925, #4929, #59, .T. ) ;
#5945=DIRECTION ( 'NONE',  ( 4.625929269271477434E-15, 1.000000000000000000, 0.000000000000000000 ) ) ;
#5959=ORIENTED_EDGE ( 'NONE', *, *, #13196, .T. ) ;
#5961=DIRECTION ( 'NONE',  ( 1.000000000000000000, 2.312964634635756072E-15, 0.000000000000000000 ) ) ;
#5962=ORIENTED_EDGE ( 'NONE', *, *, #16707, .T. ) ;
#5969=VECTOR ( 'NONE', #9488, 1000.000000000000000 ) ;
#5972=CARTESIAN_POINT ( 'NONE',  ( 14.50000000000001243, -18.49999999999999645, 4.000000000000000000 ) ) ;
#5988=CARTESIAN_POINT ( 'NONE',  ( 12.00000000000000178, -26.50000000000000355, 1.000000000000000000 ) ) ;
#5989=VECTOR ( 'NONE', #5374, 1000.000000000000000 ) ;
#6003=VERTEX_POINT ( 'NONE', #3196 ) ;
#6013=ORIENTED_EDGE ( 'NONE', *, *, #6264, .T. ) ;
#6014=VERTEX_POINT ( 'NONE', #1424 ) ;
#6017=ORIENTED_EDGE ( 'NONE', *, *, #18921, .F. ) ;
#6032=DIRECTION ( 'NONE',  ( 0.000000000000000000, 0.000000000000000000, -1.000000000000000000 ) ) ;
#6062=VECTOR ( 'NONE', #17811, 1000.000000000000000 ) ;
#6063=ORIENTED_EDGE ( 'NONE', *, *, #16145, .F. ) ;
#6069=FACE_OUTER_BOUND ( 'NONE', #17969, .T. ) ;
#6076=DIRECTION ( 'NONE',  ( -0.000000000000000000, -0.000000000000000000, -1.000000000000000000 ) ) ;
#6099=CARTESIAN_POINT ( 'NONE',  ( 15.00000000000001421, -29.99999999999998579, 1.000000000000000000 ) ) ;
#6141=EDGE_LOOP ( 'NONE', ( #19348, #6633, #13061, #5210, #8102, #216 ) ) ;
#6150=ADVANCED_FACE ( 'NONE', ( #12826 ), #15858, .F. ) ;
#6151=APPLICATION_CONTEXT ( 'automotive_design' ) ;
#6152=VERTEX_POINT ( 'NONE', #3113 ) ;
#6156=PLANE ( 'NONE',  #19684 ) ;
#6168=ORIENTED_EDGE ( 'NONE', *, *, #16852, .T. ) ;
#6179=ADVANCED_FACE ( 'NONE', ( #9691 ), #4879, .F. ) ;
#6195=CARTESIAN_POINT ( 'NONE',  ( -4.000000000000000000, 0.000000000000000000, 0.000000000000000000 ) ) ;
#6229=CARTESIAN_POINT ( 'NONE',  ( -4.000000000000000000, -8.500000000000000000, 2.392927049865408495 ) ) ;
#6258=ORIENTED_EDGE ( 'NONE', *, *, #4317, .F. ) ;
#6264=EDGE_CURVE ( 'NONE', #15518, #5711, #9584, .T. ) ;
#6284=VECTOR ( 'NONE', #3836, 1000.000000000000000 ) ;
#6285=ORIENTED_EDGE ( 'NONE', *, *, #6337, .F. ) ;
#6294=DIRECTION ( 'NONE',  ( -1.000000000000000000, 0.000000000000000000, 0.000000000000000000 ) ) ;
#6313=VECTOR ( 'NONE', #15866, 1000.000000000000000 ) ;
#6317=CARTESIAN_POINT ( 'NONE',  ( -9.999999999999998224, -30.00000000000000355, 0.000000000000000000 ) ) ;
#6322=EDGE_CURVE ( 'NONE', #13949, #6936, #7279, .T. ) ;
#6334=AXIS2_PLACEMENT_3D ( 'NONE', #15930, #1412, #46 ) ;
#6337=EDGE_CURVE ( 'NONE', #12047, #13360, #794, .T. ) ;
#6345=EDGE_CURVE ( 'NONE', #6014, #18185, #9757, .T. ) ;
#6354=EDGE_CURVE ( 'NONE', #6936, #3922, #2056, .T. ) ;
#6357=ORIENTED_EDGE ( 'NONE', *, *, #9821, .T. ) ;
#6387=DIRECTION ( 'NONE',  ( 0.000000000000000000, 0.2588190451025245697, 0.9659258262890673130 ) ) ;
#6391=DIRECTION ( 'NONE',  ( -4.625929269271486111E-15, -1.000000000000000000, 0.000000000000000000 ) ) ;
#6407=ORIENTED_EDGE ( 'NONE', *, *, #20532, .F. ) ;
#6409=CARTESIAN_POINT ( 'NONE',  ( -12.00000000000000000, -25.49999999999998934, 4.000000000000000000 ) ) ;
#6418=EDGE_CURVE ( 'NONE', #4642, #15518, #18677, .T. ) ;
#6419=DIRECTION ( 'NONE',  ( -0.000000000000000000, -0.000000000000000000, -1.000000000000000000 ) ) ;
#6435=VECTOR ( 'NONE', #11567, 1000.000000000000000 ) ;
#6453=AXIS2_PLACEMENT_3D ( 'NONE', #5787, #18547, #1284 ) ;
#6465=AXIS2_PLACEMENT_3D ( 'NONE', #15151, #18095, #18193 ) ;
#6473=DIRECTION ( 'NONE',  ( 1.000000000000000000, 6.938893903907222067E-15, 0.000000000000000000 ) ) ;
#6488=FACE_OUTER_BOUND ( 'NONE', #7559, .T. ) ;
#6521=CARTESIAN_POINT ( 'NONE',  ( -5.000000000000000000, -12.50000000000000000, 4.500000000000000888 ) ) ;
#6572=VERTEX_POINT ( 'NONE', #15933 ) ;
#6607=ORIENTED_EDGE ( 'NONE', *, *, #10917, .T. ) ;
#6625=CARTESIAN_POINT ( 'NONE',  ( 11.99999999999999822, -17.50000000000000000, 1.000000000000000000 ) ) ;
#6633=ORIENTED_EDGE ( 'NONE', *, *, #16068, .F. ) ;
#6640=CARTESIAN_POINT ( 'NONE',  ( -14.49999999999999645, -21.00000000000000355, 4.000000000000000000 ) ) ;
#6643=DIRECTION ( 'NONE',  ( 0.000000000000000000, 0.000000000000000000, 1.000000000000000000 ) ) ;
#6659=VERTEX_POINT ( 'NONE', #14981 ) ;
#6674=EDGE_CURVE ( 'NONE', #4492, #2477, #19512, .T. ) ;
#6697=( GEOMETRIC_REPRESENTATION_CONTEXT ( 3 ) GLOBAL_UNCERTAINTY_ASSIGNED_CONTEXT ( ( #16960 ) ) GLOBAL_UNIT_ASSIGNED_CONTEXT ( ( #14952, #10252, #4084 ) ) REPRESENTATION_CONTEXT ( 'NONE', 'WORKASPACE' ) );
#6703=VECTOR ( 'NONE', #19418, 1000.000000000000000 ) ;
#6705=DIRECTION ( 'NONE',  ( 1.000000000000000000, 2.312964634635731617E-15, 0.000000000000000000 ) ) ;
#6709=EDGE_LOOP ( 'NONE', ( #4232, #329, #5496, #14812 ) ) ;
#6716=LINE ( 'NONE', #19581, #12114 ) ;
#6723=FACE_BOUND ( 'NONE', #14823, .T. ) ;
#6754=CARTESIAN_POINT ( 'NONE',  ( -14.49999999999999645, -21.00000000000000355, 1.000000000000000000 ) ) ;
#6757=ORIENTED_EDGE ( 'NONE', *, *, #18090, .F. ) ;
#6767=AXIS2_PLACEMENT_3D ( 'NONE', #386, #19325, #14704 ) ;
#6771=EDGE_LOOP ( 'NONE', ( #1414, #13488, #8380, #10223 ) ) ;
#6773=CARTESIAN_POINT ( 'NONE',  ( 14.50000000000000000, -20.99999999999998934, 1.000000000000000000 ) ) ;
#6786=EDGE_CURVE ( 'NONE', #14414, #17290, #10081, .T. ) ;
#6791=ORIENTED_EDGE ( 'NONE', *, *, #150, .F. ) ;
#6806=ADVANCED_FACE ( 'NONE', ( #8719 ), #10280, .F. ) ;
#6812=CARTESIAN_POINT ( 'NONE',  ( -7.500000000000000888, -9.999999999999992895, 2.500000000000000000 ) ) ;
#6814=LINE ( 'NONE', #14651, #17473 ) ;
#6847=DIRECTION ( 'NONE',  ( -1.000000000000000000, 6.938893903907222067E-15, 0.000000000000000000 ) ) ;
#6850=EDGE_LOOP ( 'NONE', ( #526, #8361, #3185, #13108 ) ) ;
#6860=ORIENTED_EDGE ( 'NONE', *, *, #9410, .T. ) ;
#6863=VERTEX_POINT ( 'NONE', #6099 ) ;
#6868=EDGE_CURVE ( 'NONE', #20635, #9650, #10701, .T. ) ;
#6873=CARTESIAN_POINT ( 'NONE',  ( -15.49999999999999822, -22.99999999999999289, 4.000000000000000000 ) ) ;
#6894=AXIS2_PLACEMENT_3D ( 'NONE', #13588, #9202, #20411 ) ;
#6917=( GEOMETRIC_REPRESENTATION_CONTEXT ( 3 ) GLOBAL_UNCERTAINTY_ASSIGNED_CONTEXT ( ( #1282 ) ) GLOBAL_UNIT_ASSIGNED_CONTEXT ( ( #8702, #16748, #7238 ) ) REPRESENTATION_CONTEXT ( 'NONE', 'WORKASPACE' ) );
#6936=VERTEX_POINT ( 'NONE', #5988 ) ;
#6940=EDGE_CURVE ( 'NONE', #3190, #1434, #8826, .T. ) ;
#6946=VECTOR ( 'NONE', #603, 1000.000000000000000 ) ;
#6963=VECTOR ( 'NONE', #19028, 1000.000000000000000 ) ;
#6970=LINE ( 'NONE', #6773, #7663 ) ;
#6972=EDGE_CURVE ( 'NONE', #5711, #7723, #10494, .T. ) ;
#6991=EDGE_LOOP ( 'NONE', ( #3379, #5389, #2714, #3963 ) ) ;
#6993=AXIS2_PLACEMENT_3D ( 'NONE', #8446, #17952, #10004 ) ;
#7010=FACE_OUTER_BOUND ( 'NONE', #6771, .T. ) ;
#7016=LINE ( 'NONE', #18305, #8996 ) ;
#7021=( NAMED_UNIT ( * ) PLANE_ANGLE_UNIT ( ) SI_UNIT ( $, .RADIAN. ) );
#7023=CARTESIAN_POINT ( 'NONE',  ( 7.500000000000002665, -9.999999999999991118, 1.000000000000000000 ) ) ;
#7024=VECTOR ( 'NONE', #18509, 1000.000000000000000 ) ;
#7030=VECTOR ( 'NONE', #7501, 1000.000000000000000 ) ;
#7050=PLANE ( 'NONE',  #18609 ) ;
#7051=ADVANCED_FACE ( 'NONE', ( #967 ), #9227, .T. ) ;
#7068=VERTEX_POINT ( 'NONE', #7463 ) ;
#7070=DIRECTION ( 'NONE',  ( 1.000000000000000000, 2.312964634635730039E-15, 0.000000000000000000 ) ) ;
#7091=AXIS2_PLACEMENT_3D ( 'NONE', #8330, #1947, #3311 ) ;
#7097=DIRECTION ( 'NONE',  ( 0.000000000000000000, 0.000000000000000000, 1.000000000000000000 ) ) ;
#7126=ADVANCED_FACE ( 'NONE', ( #18962 ), #11309, .F. ) ;
#7164=DIRECTION ( 'NONE',  ( -1.000000000000000000, 6.938893903907222067E-15, 0.000000000000000000 ) ) ;
#7191=LINE ( 'NONE', #13765, #523 ) ;
#7221=DIRECTION ( 'NONE',  ( -0.000000000000000000, -0.000000000000000000, -1.000000000000000000 ) ) ;
#7231=CYLINDRICAL_SURFACE ( 'NONE', #9256, 1.499999999999999556 ) ;
#7238=( NAMED_UNIT ( * ) SI_UNIT ( $, .STERADIAN. ) SOLID_ANGLE_UNIT ( ) );
#7242=DIRECTION ( 'NONE',  ( -5.204170427930411817E-15, 1.000000000000000000, 0.000000000000000000 ) ) ;
#7246=VERTEX_POINT ( 'NONE', #7023 ) ;
#7276=EDGE_CURVE ( 'NONE', #17965, #11896, #6716, .T. ) ;
#7279=LINE ( 'NONE', #486, #6435 ) ;
#7308=ADVANCED_FACE ( 'NONE', ( #8489 ), #11613, .T. ) ;
#7312=EDGE_CURVE ( 'NONE', #13849, #20560, #18115, .T. ) ;
#7338=DIRECTION ( 'NONE',  ( -6.938893903907232322E-16, 1.000000000000000000, 0.000000000000000000 ) ) ;
#7369=DIRECTION ( 'NONE',  ( -0.000000000000000000, -0.000000000000000000, -1.000000000000000000 ) ) ;
#7387=EDGE_CURVE ( 'NONE', #5651, #13228, #6814, .T. ) ;
#7401=CARTESIAN_POINT ( 'NONE',  ( -14.49999999999999645, -22.99999999999998579, 1.000000000000000000 ) ) ;
#7414=ORIENTED_EDGE ( 'NONE', *, *, #6322, .T. ) ;
#7417=ORIENTED_EDGE ( 'NONE', *, *, #3262, .F. ) ;
#7421=CARTESIAN_POINT ( 'NONE',  ( -9.000000000000000000, -9.999999999999992895, 2.500000000000000000 ) ) ;
#7441=VERTEX_POINT ( 'NONE', #3566 ) ;
#7451=EDGE_CURVE ( 'NONE', #20560, #551, #9946, .T. ) ;
#7463=CARTESIAN_POINT ( 'NONE',  ( -14.49999999999999645, -22.99999999999998579, 4.000000000000000000 ) ) ;
#7472=EDGE_CURVE ( 'NONE', #6152, #11135, #846, .T. ) ;
#7492=ORIENTED_EDGE ( 'NONE', *, *, #19595, .T. ) ;
#7497=DIRECTION ( 'NONE',  ( 0.000000000000000000, 1.000000000000000000, -0.000000000000000000 ) ) ;
#7501=DIRECTION ( 'NONE',  ( 5.204170427930411817E-15, -1.000000000000000000, 0.000000000000000000 ) ) ;
#7511=ORIENTED_EDGE ( 'NONE', *, *, #8347, .F. ) ;
#7521=CARTESIAN_POINT ( 'NONE',  ( 15.00000000000001599, -18.49999999999999645, 4.000000000000000000 ) ) ;
#7540=EDGE_CURVE ( 'NONE', #3927, #20096, #16156, .T. ) ;
#7559=EDGE_LOOP ( 'NONE', ( #18202, #14334, #8081, #19198, #15646, #10311 ) ) ;
#7660=VERTEX_POINT ( 'NONE', #13801 ) ;
#7663=VECTOR ( 'NONE', #17856, 1000.000000000000000 ) ;
#7669=CARTESIAN_POINT ( 'NONE',  ( 14.50000000000000000, -23.00000000000001421, 4.000000000000000000 ) ) ;
#7703=DIRECTION ( 'NONE',  ( 0.000000000000000000, 0.000000000000000000, -1.000000000000000000 ) ) ;
#7712=CARTESIAN_POINT ( 'NONE',  ( 5.000000000000000000, -12.50000000000000000, 4.500000000000000888 ) ) ;
#7719=EDGE_CURVE ( 'NONE', #19250, #4026, #1562, .T. ) ;
#7720=VECTOR ( 'NONE', #16178, 1000.000000000000000 ) ;
#7723=VERTEX_POINT ( 'NONE', #1367 ) ;
#7728=LINE ( 'NONE', #3019, #11306 ) ;
#7746=ORIENTED_EDGE ( 'NONE', *, *, #16689, .F. ) ;
#7749=EDGE_CURVE ( 'NONE', #9890, #5036, #9607, .T. ) ;
#7759=EDGE_CURVE ( 'NONE', #18720, #4492, #14307, .T. ) ;
#7781=CARTESIAN_POINT ( 'NONE',  ( -15.49999999999999822, -22.99999999999999289, 1.000000000000000000 ) ) ;
#7794=ORIENTED_EDGE ( 'NONE', *, *, #18860, .T. ) ;
#7809=CARTESIAN_POINT ( 'NONE',  ( -11.99999999999999467, -17.50000000000000000, 4.000000000000000000 ) ) ;
#7818=CARTESIAN_POINT ( 'NONE',  ( -27.00000000000000000, 0.000000000000000000, 1.000000000000000000 ) ) ;
#7839=FACE_OUTER_BOUND ( 'NONE', #8106, .T. ) ;
#7844=CARTESIAN_POINT ( 'NONE',  ( 15.50000000000000178, -20.99999999999999645, 4.000000000000000000 ) ) ;
#7848=ADVANCED_FACE ( 'NONE', ( #6488 ), #12850, .F. ) ;
#7867=DIRECTION ( 'NONE',  ( -1.000000000000000000, -2.312964634635731617E-15, 0.000000000000000000 ) ) ;
#7883=DIRECTION ( 'NONE',  ( -0.000000000000000000, -0.000000000000000000, -1.000000000000000000 ) ) ;
#7945=DIRECTION ( 'NONE',  ( -1.000000000000000000, 4.625929269271486111E-15, 0.000000000000000000 ) ) ;
#7959=AXIS2_PLACEMENT_3D ( 'NONE', #12218, #4484, #5943 ) ;
#7960=EDGE_LOOP ( 'NONE', ( #10674, #8381, #9173, #14159, #13876, #11131, #15164, #4500 ) ) ;
#7974=PLANE ( 'NONE',  #9079 ) ;
#7977=ORIENTED_EDGE ( 'NONE', *, *, #7540, .F. ) ;
#7985=AXIS2_PLACEMENT_3D ( 'NONE', #7421, #9088, #18292 ) ;
#7994=VECTOR ( 'NONE', #8752, 1000.000000000000000 ) ;
#8003=DIRECTION ( 'NONE',  ( 0.000000000000000000, 0.000000000000000000, 1.000000000000000000 ) ) ;
#8023=DIRECTION ( 'NONE',  ( 3.469446951953619119E-16, 1.000000000000000000, -0.000000000000000000 ) ) ;
#8033=DIRECTION ( 'NONE',  ( 1.000000000000000000, 0.000000000000000000, -0.000000000000000000 ) ) ;
#8036=VECTOR ( 'NONE', #11901, 1000.000000000000000 ) ;
#8050=CARTESIAN_POINT ( 'NONE',  ( -4.999999999999997335, -7.500000000000000000, 1.000000000000000000 ) ) ;
#8081=ORIENTED_EDGE ( 'NONE', *, *, #14525, .F. ) ;
#8102=ORIENTED_EDGE ( 'NONE', *, *, #3407, .T. ) ;
#8106=EDGE_LOOP ( 'NONE', ( #18299, #15927, #13324, #7794 ) ) ;
#8123=VECTOR ( 'NONE', #12364, 1000.000000000000000 ) ;
#8132=ORIENTED_EDGE ( 'NONE', *, *, #16852, .F. ) ;
#8149=ORIENTED_EDGE ( 'NONE', *, *, #13568, .F. ) ;
#8180=DIRECTION ( 'NONE',  ( 1.000000000000000000, 0.000000000000000000, 0.000000000000000000 ) ) ;
#8185=DIRECTION ( 'NONE',  ( 0.000000000000000000, 0.000000000000000000, 1.000000000000000000 ) ) ;
#8198=AXIS2_PLACEMENT_3D ( 'NONE', #11342, #9567, #4760 ) ;
#8216=CARTESIAN_POINT ( 'NONE',  ( -4.000000000000000000, -12.50000000000000000, 3.464723819589916154 ) ) ;
#8221=ORIENTED_EDGE ( 'NONE', *, *, #10000, .T. ) ;
#8248=EDGE_LOOP ( 'NONE', ( #12616, #9706, #5886, #8941 ) ) ;
#8268=CARTESIAN_POINT ( 'NONE',  ( -15.49999999999999822, -22.99999999999999289, 4.000000000000000000 ) ) ;
#8301=ORIENTED_EDGE ( 'NONE', *, *, #2501, .F. ) ;
#8302=ORIENTED_EDGE ( 'NONE', *, *, #13952, .T. ) ;
#8311=DIRECTION ( 'NONE',  ( -6.938893903907222067E-15, 1.000000000000000000, 0.000000000000000000 ) ) ;
#8326=ORIENTED_EDGE ( 'NONE', *, *, #13695, .T. ) ;
#8330=CARTESIAN_POINT ( 'NONE',  ( -5.000000000000000000, 0.000000000000000000, 0.000000000000000000 ) ) ;
#8347=EDGE_CURVE ( 'NONE', #7660, #19894, #247, .T. ) ;
#8361=ORIENTED_EDGE ( 'NONE', *, *, #4002, .F. ) ;
#8368=LINE ( 'NONE', #19158, #452 ) ;
#8380=ORIENTED_EDGE ( 'NONE', *, *, #10196, .F. ) ;
#8381=ORIENTED_EDGE ( 'NONE', *, *, #15654, .F. ) ;
#8393=AXIS2_PLACEMENT_3D ( 'NONE', #4196, #15275, #4408 ) ;
#8404=ADVANCED_FACE ( 'NONE', ( #16764 ), #8613, .F. ) ;
#8440=ADVANCED_FACE ( 'NONE', ( #15193 ), #7050, .F. ) ;
#8446=CARTESIAN_POINT ( 'NONE',  ( 5.000000000000000000, -7.500000000000000000, 1.000000000000000000 ) ) ;
#8456=VERTEX_POINT ( 'NONE', #8513 ) ;
#8461=CARTESIAN_POINT ( 'NONE',  ( -9.999999999999996447, -34.99999999999999289, 1.000000000000000000 ) ) ;
#8464=VECTOR ( 'NONE', #2104, 1000.000000000000227 ) ;
#8489=FACE_OUTER_BOUND ( 'NONE', #13544, .T. ) ;
#8491=CARTESIAN_POINT ( 'NONE',  ( 14.50000000000000000, -23.00000000000001421, 4.000000000000000000 ) ) ;
#8513=CARTESIAN_POINT ( 'NONE',  ( 10.49999999999999645, -9.999999999999991118, 2.500000000000000000 ) ) ;
#8574=EDGE_CURVE ( 'NONE', #11223, #12439, #1900, .T. ) ;
#8582=ADVANCED_FACE ( 'NONE', ( #15909 ), #1799, .F. ) ;
#8584=FILL_AREA_STYLE_COLOUR ( '', #17361 ) ;
#8605=ADVANCED_FACE ( 'NONE', ( #14654 ), #11012, .F. ) ;
#8610=ORIENTED_EDGE ( 'NONE', *, *, #13196, .F. ) ;
#8613=PLANE ( 'NONE',  #15921 ) ;
#8620=EDGE_CURVE ( 'NONE', #17290, #13360, #9439, .T. ) ;
#8632=PLANE ( 'NONE',  #9711 ) ;
#8641=DIRECTION ( 'NONE',  ( -1.000000000000000000, 4.625929269271477434E-15, 0.000000000000000000 ) ) ;
#8654=EDGE_LOOP ( 'NONE', ( #10174, #12692, #20248, #13140 ) ) ;
#8675=AXIS2_PLACEMENT_3D ( 'NONE', #10210, #8641, #19540 ) ;
#8684=CIRCLE ( 'NONE', #10355, 1.499999999999998668 ) ;
#8702=( LENGTH_UNIT ( ) NAMED_UNIT ( * ) SI_UNIT ( .MILLI., .METRE. ) );
#8715=ORIENTED_EDGE ( 'NONE', *, *, #4677, .F. ) ;
#8719=FACE_OUTER_BOUND ( 'NONE', #7960, .T. ) ;
#8724=ADVANCED_FACE ( 'NONE', ( #19997 ), #7231, .T. ) ;
#8729=EDGE_CURVE ( 'NONE', #4492, #16474, #14011, .T. ) ;
#8746=DIRECTION ( 'NONE',  ( 1.000000000000000000, -6.938893903907222067E-15, 0.000000000000000000 ) ) ;
#8752=DIRECTION ( 'NONE',  ( 0.000000000000000000, 1.000000000000000000, 0.000000000000000000 ) ) ;
#8760=CARTESIAN_POINT ( 'NONE',  ( 15.50000000000001776, -17.49999999999999645, 4.000000000000000000 ) ) ;
#8802=CARTESIAN_POINT ( 'NONE',  ( -9.000000000000000000, -9.999999999999992895, 1.000000000000000000 ) ) ;
#8803=DIRECTION ( 'NONE',  ( -1.000000000000000000, -2.312964634635731617E-15, 0.000000000000000000 ) ) ;
#8826=LINE ( 'NONE', #2752, #15786 ) ;
#8837=ORIENTED_EDGE ( 'NONE', *, *, #13743, .F. ) ;
#8840=ADVANCED_FACE ( 'NONE', ( #17669 ), #14423, .T. ) ;
#8860=DIRECTION ( 'NONE',  ( -1.000000000000000000, -0.000000000000000000, -0.000000000000000000 ) ) ;
#8866=EDGE_LOOP ( 'NONE', ( #9918, #12951, #13641, #5962 ) ) ;
#8870=LINE ( 'NONE', #15240, #1601 ) ;
#8889=CARTESIAN_POINT ( 'NONE',  ( -4.000000000000000000, -12.50000000000000000, 3.464723819589916154 ) ) ;
#8890=DIRECTION ( 'NONE',  ( 1.000000000000000000, 3.469446951953619119E-16, -0.000000000000000000 ) ) ;
#8900=DIRECTION ( 'NONE',  ( 0.000000000000000000, 0.000000000000000000, 1.000000000000000000 ) ) ;
#8918=LINE ( 'NONE', #18544, #20386 ) ;
#8919=VERTEX_POINT ( 'NONE', #3547 ) ;
#8941=ORIENTED_EDGE ( 'NONE', *, *, #10313, .T. ) ;
#8946=ORIENTED_EDGE ( 'NONE', *, *, #6940, .F. ) ;
#8971=ORIENTED_EDGE ( 'NONE', *, *, #14251, .T. ) ;
#8993=VECTOR ( 'NONE', #14683, 1000.000000000000000 ) ;
#8996=VECTOR ( 'NONE', #7221, 1000.000000000000000 ) ;
#9006=DIRECTION ( 'NONE',  ( 4.625929269271486900E-15, 1.000000000000000000, 0.000000000000000000 ) ) ;
#9025=MECHANICAL_DESIGN_GEOMETRIC_PRESENTATION_REPRESENTATION('',(#20054),#6697);
#9046=VECTOR ( 'NONE', #8803, 1000.000000000000000 ) ;
#9051=CARTESIAN_POINT ( 'NONE',  ( 14.50000000000000000, -23.00000000000001421, 4.000000000000000000 ) ) ;
#9054=FACE_OUTER_BOUND ( 'NONE', #19378, .T. ) ;
#9058=AXIS2_PLACEMENT_3D ( 'NONE', #8268, #14748, #212 ) ;
#9061=CARTESIAN_POINT ( 'NONE',  ( 11.99999999999999822, -17.50000000000000000, 4.000000000000000000 ) ) ;
#9079=AXIS2_PLACEMENT_3D ( 'NONE', #11220, #17596, #11122 ) ;
#9088=DIRECTION ( 'NONE',  ( 0.000000000000000000, 0.000000000000000000, 1.000000000000000000 ) ) ;
#9101=ORIENTED_EDGE ( 'NONE', *, *, #2777, .T. ) ;
#9106=VECTOR ( 'NONE', #17100, 1000.000000000000000 ) ;
#9127=DIRECTION ( 'NONE',  ( 1.000000000000000000, 2.312964634635730039E-15, 0.000000000000000000 ) ) ;
#9164=FACE_OUTER_BOUND ( 'NONE', #4750, .T. ) ;
#9173=ORIENTED_EDGE ( 'NONE', *, *, #10917, .F. ) ;
#9185=FACE_OUTER_BOUND ( 'NONE', #11874, .T. ) ;
#9202=DIRECTION ( 'NONE',  ( 0.000000000000000000, 0.000000000000000000, 1.000000000000000000 ) ) ;
#9209=CARTESIAN_POINT ( 'NONE',  ( 15.50000000000000178, -20.99999999999999645, 1.000000000000000000 ) ) ;
#9219=EDGE_CURVE ( 'NONE', #13278, #13849, #1647, .T. ) ;
#9227=PLANE ( 'NONE',  #6453 ) ;
#9250=EDGE_LOOP ( 'NONE', ( #14002, #3509, #8326, #2906 ) ) ;
#9256=AXIS2_PLACEMENT_3D ( 'NONE', #849, #5869, #13698 ) ;
#9263=DIRECTION ( 'NONE',  ( 1.000000000000000000, 0.000000000000000000, 0.000000000000000000 ) ) ;
#9288=VECTOR ( 'NONE', #20164, 1000.000000000000227 ) ;
#9301=DIRECTION ( 'NONE',  ( -2.312964634635756072E-15, 1.000000000000000000, 0.000000000000000000 ) ) ;
#9302=ORIENTED_EDGE ( 'NONE', *, *, #14474, .F. ) ;
#9316=VECTOR ( 'NONE', #2030, 1000.000000000000000 ) ;
#9355=EDGE_CURVE ( 'NONE', #18598, #12925, #10962, .T. ) ;
#9394=DIRECTION ( 'NONE',  ( 0.000000000000000000, 0.000000000000000000, 1.000000000000000000 ) ) ;
#9401=VECTOR ( 'NONE', #9447, 1000.000000000000000 ) ;
#9404=CARTESIAN_POINT ( 'NONE',  ( -9.999999999999998224, -30.00000000000000355, 0.000000000000000000 ) ) ;
#9410=EDGE_CURVE ( 'NONE', #9650, #19732, #14601, .T. ) ;
#9415=CARTESIAN_POINT ( 'NONE',  ( -15.49999999999999822, -22.99999999999999289, 4.000000000000000000 ) ) ;
#9423=ADVANCED_FACE ( 'NONE', ( #5402 ), #14911, .F. ) ;
#9432=VERTEX_POINT ( 'NONE', #11774 ) ;
#9436=ORIENTED_EDGE ( 'NONE', *, *, #13064, .F. ) ;
#9439=LINE ( 'NONE', #1489, #14937 ) ;
#9441=LINE ( 'NONE', #3067, #2671 ) ;
#9443=EDGE_CURVE ( 'NONE', #6572, #18339, #20365, .T. ) ;
#9447=DIRECTION ( 'NONE',  ( 1.000000000000000000, -2.312964634635752916E-15, 0.000000000000000000 ) ) ;
#9456=ORIENTED_EDGE ( 'NONE', *, *, #2878, .T. ) ;
#9462=ORIENTED_EDGE ( 'NONE', *, *, #18596, .F. ) ;
#9476=LINE ( 'NONE', #19001, #10717 ) ;
#9488=DIRECTION ( 'NONE',  ( 4.625929269271486900E-15, 1.000000000000000000, 0.000000000000000000 ) ) ;
#9495=LINE ( 'NONE', #18919, #17374 ) ;
#9496=LINE ( 'NONE', #12832, #18331 ) ;
#9517=EDGE_CURVE ( 'NONE', #2477, #2500, #6970, .T. ) ;
#9542=ADVANCED_FACE ( 'NONE', ( #18165 ), #3424, .T. ) ;
#9546=CYLINDRICAL_SURFACE ( 'NONE', #5378, 59.99999999999999289 ) ;
#9567=DIRECTION ( 'NONE',  ( 2.312964634635752916E-15, 1.000000000000000000, -0.000000000000000000 ) ) ;
#9584=LINE ( 'NONE', #1642, #3089 ) ;
#9606=EDGE_CURVE ( 'NONE', #12439, #4026, #5818, .T. ) ;
#9607=LINE ( 'NONE', #9415, #15129 ) ;
#9627=EDGE_LOOP ( 'NONE', ( #1951, #6017, #18212, #12993 ) ) ;
#9640=CARTESIAN_POINT ( 'NONE',  ( -15.49999999999998224, -17.49999999999999645, 4.000000000000000000 ) ) ;
#9641=VECTOR ( 'NONE', #7164, 1000.000000000000000 ) ;
#9650=VERTEX_POINT ( 'NONE', #11977 ) ;
#9671=PLANE ( 'NONE',  #8198 ) ;
#9691=FACE_OUTER_BOUND ( 'NONE', #3728, .T. ) ;
#9706=ORIENTED_EDGE ( 'NONE', *, *, #9606, .F. ) ;
#9711=AXIS2_PLACEMENT_3D ( 'NONE', #16984, #20147, #7070 ) ;
#9745=AXIS2_PLACEMENT_3D ( 'NONE', #1151, #8890, #10772 ) ;
#9746=EDGE_LOOP ( 'NONE', ( #2383, #2976, #20352, #20277, #18412, #1155 ) ) ;
#9757=CIRCLE ( 'NONE', #745, 59.99999999999998579 ) ;
#9821=EDGE_CURVE ( 'NONE', #10023, #12236, #3191, .T. ) ;
#9849=LINE ( 'NONE', #4647, #19892 ) ;
#9870=AXIS2_PLACEMENT_3D ( 'NONE', #14193, #20600, #19138 ) ;
#9881=LINE ( 'NONE', #1832, #19009 ) ;
#9890=VERTEX_POINT ( 'NONE', #3093 ) ;
#9895=CARTESIAN_POINT ( 'NONE',  ( -4.000000000000000000, -8.500000000000000000, 2.392927049865408495 ) ) ;
#9901=CARTESIAN_POINT ( 'NONE',  ( -9.000000000000000000, -9.999999999999992895, 2.500000000000000000 ) ) ;
#9914=EDGE_LOOP ( 'NONE', ( #9101, #1845 ) ) ;
#9918=ORIENTED_EDGE ( 'NONE', *, *, #13616, .F. ) ;
#9923=ORIENTED_EDGE ( 'NONE', *, *, #1990, .F. ) ;
#9927=AXIS2_PLACEMENT_3D ( 'NONE', #1565, #1776, #19049 ) ;
#9941=ORIENTED_EDGE ( 'NONE', *, *, #14525, .T. ) ;
#9946=LINE ( 'NONE', #19680, #8464 ) ;
#9957=VECTOR ( 'NONE', #16583, 1000.000000000000000 ) ;
#9969=DIRECTION ( 'NONE',  ( 1.000000000000000000, -2.312964634635752916E-15, 0.000000000000000000 ) ) ;
#9975=LINE ( 'NONE', #16356, #8993 ) ;
#10000=EDGE_CURVE ( 'NONE', #4871, #6936, #9441, .T. ) ;
#10004=DIRECTION ( 'NONE',  ( 0.000000000000000000, -0.000000000000000000, -1.000000000000000000 ) ) ;
#10007=LINE ( 'NONE', #5294, #17675 ) ;
#10023=VERTEX_POINT ( 'NONE', #9640 ) ;
#10044=DIRECTION ( 'NONE',  ( -1.000000000000000000, -6.938893903907232322E-16, 0.000000000000000000 ) ) ;
#10055=AXIS2_PLACEMENT_3D ( 'NONE', #5129, #5225, #10044 ) ;
#10058=EDGE_CURVE ( 'NONE', #14903, #13849, #14450, .T. ) ;
#10063=FACE_BOUND ( 'NONE', #6141, .T. ) ;
#10072=AXIS2_PLACEMENT_3D ( 'NONE', #4300, #10581, #5875 ) ;
#10081=LINE ( 'NONE', #5370, #1432 ) ;
#10082=EDGE_CURVE ( 'NONE', #13278, #18598, #5431, .T. ) ;
#10084=LINE ( 'NONE', #6640, #14303 ) ;
#10104=ORIENTED_EDGE ( 'NONE', *, *, #5944, .T. ) ;
#10110=EDGE_CURVE ( 'NONE', #8456, #6003, #15150, .T. ) ;
#10111=CARTESIAN_POINT ( 'NONE',  ( 9.000000000000000000, -9.999999999999991118, 2.500000000000000000 ) ) ;
#10116=CARTESIAN_POINT ( 'NONE',  ( 15.00000000000001421, -29.99999999999998579, 1.000000000000000000 ) ) ;
#10134=CARTESIAN_POINT ( 'NONE',  ( 14.50000000000000000, -23.00000000000001421, 4.000000000000000000 ) ) ;
#10157=VECTOR ( 'NONE', #3548, 1000.000000000000000 ) ;
#10174=ORIENTED_EDGE ( 'NONE', *, *, #6345, .T. ) ;
#10180=DIRECTION ( 'NONE',  ( -1.000000000000000000, 6.938893903907222067E-15, 0.000000000000000000 ) ) ;
#10181=DIRECTION ( 'NONE',  ( 0.000000000000000000, -0.000000000000000000, -1.000000000000000000 ) ) ;
#10184=CARTESIAN_POINT ( 'NONE',  ( 14.50000000000001243, -18.49999999999999645, 4.000000000000000000 ) ) ;
#10196=EDGE_CURVE ( 'NONE', #1434, #6863, #15353, .T. ) ;
#10210=CARTESIAN_POINT ( 'NONE',  ( -15.49999999999999822, -20.99999999999999645, 4.000000000000000000 ) ) ;
#10211=DIRECTION ( 'NONE',  ( -0.000000000000000000, -0.000000000000000000, -1.000000000000000000 ) ) ;
#10223=ORIENTED_EDGE ( 'NONE', *, *, #14932, .T. ) ;
#10252=( NAMED_UNIT ( * ) PLANE_ANGLE_UNIT ( ) SI_UNIT ( $, .RADIAN. ) );
#10255=ADVANCED_FACE ( 'NONE', ( #3955 ), #1035, .T. ) ;
#10261=CARTESIAN_POINT ( 'NONE',  ( -14.99999999999999645, -30.00000000000000711, 1.000000000000000000 ) ) ;
#10280=PLANE ( 'NONE',  #10797 ) ;
#10301=ADVANCED_FACE ( 'NONE', ( #9185 ), #6156, .T. ) ;
#10306=ORIENTED_EDGE ( 'NONE', *, *, #18217, .F. ) ;
#10311=ORIENTED_EDGE ( 'NONE', *, *, #18090, .T. ) ;
#10313=EDGE_CURVE ( 'NONE', #11223, #16474, #11170, .T. ) ;
#10355=AXIS2_PLACEMENT_3D ( 'NONE', #19109, #8003, #2813 ) ;
#10358=ORIENTED_EDGE ( 'NONE', *, *, #10000, .F. ) ;
#10384=ORIENTED_EDGE ( 'NONE', *, *, #7312, .T. ) ;
#10400=FACE_OUTER_BOUND ( 'NONE', #10447, .T. ) ;
#10401=VECTOR ( 'NONE', #2337, 1000.000000000000000 ) ;
#10421=VECTOR ( 'NONE', #16275, 1000.000000000000000 ) ;
#10426=EDGE_CURVE ( 'NONE', #19461, #2483, #9495, .T. ) ;
#10440=ORIENTED_EDGE ( 'NONE', *, *, #2878, .F. ) ;
#10441=ADVANCED_FACE ( 'NONE', ( #4378 ), #10761, .F. ) ;
#10445=VERTEX_POINT ( 'NONE', #2911 ) ;
#10447=EDGE_LOOP ( 'NONE', ( #1549, #15920, #6168, #9436 ) ) ;
#10455=CARTESIAN_POINT ( 'NONE',  ( 12.00000000000000178, -18.50000000000000355, 4.000000000000000000 ) ) ;
#10474=CARTESIAN_POINT ( 'NONE',  ( 15.00000000000001421, -17.49999999999999645, 1.000000000000000000 ) ) ;
#10494=LINE ( 'NONE', #15291, #8123 ) ;
#10564=EDGE_CURVE ( 'NONE', #9890, #7068, #10007, .T. ) ;
#10581=DIRECTION ( 'NONE',  ( -1.000000000000000000, 4.625929269271486111E-15, 0.000000000000000000 ) ) ;
#10600=LINE ( 'NONE', #18659, #19351 ) ;
#10625=PLANE ( 'NONE',  #19565 ) ;
#10626=EDGE_CURVE ( 'NONE', #8919, #6152, #17181, .T. ) ;
#10628=DIRECTION ( 'NONE',  ( 1.000000000000000000, 0.000000000000000000, 0.000000000000000000 ) ) ;
#10667=LINE ( 'NONE', #14106, #642 ) ;
#10670=ORIENTED_EDGE ( 'NONE', *, *, #5944, .F. ) ;
#10674=ORIENTED_EDGE ( 'NONE', *, *, #6345, .F. ) ;
#10685=CARTESIAN_POINT ( 'NONE',  ( -14.49999999999998401, -25.49999999999999645, 4.000000000000000000 ) ) ;
#10696=VECTOR ( 'NONE', #11695, 1000.000000000000000 ) ;
#10701=LINE ( 'NONE', #12467, #757 ) ;
#10707=DIRECTION ( 'NONE',  ( 1.000000000000000000, 6.938893903907222067E-15, 0.000000000000000000 ) ) ;
#10717=VECTOR ( 'NONE', #19313, 1000.000000000000000 ) ;
#10723=EDGE_LOOP ( 'NONE', ( #12792, #17244, #1027, #2614 ) ) ;
#10736=DIRECTION ( 'NONE',  ( 2.312964634635731617E-15, -1.000000000000000000, 0.000000000000000000 ) ) ;
#10761=PLANE ( 'NONE',  #11040 ) ;
#10772=DIRECTION ( 'NONE',  ( -3.469446951953619119E-16, 1.000000000000000000, 0.000000000000000000 ) ) ;
#10797=AXIS2_PLACEMENT_3D ( 'NONE', #5260, #16762, #462 ) ;
#10819=LINE ( 'NONE', #5895, #1632 ) ;
#10841=DIRECTION ( 'NONE',  ( 0.000000000000000000, 1.000000000000000000, 0.000000000000000000 ) ) ;
#10842=DIRECTION ( 'NONE',  ( 1.000000000000000000, -2.312964634635752916E-15, 0.000000000000000000 ) ) ;
#10843=FACE_OUTER_BOUND ( 'NONE', #8248, .T. ) ;
#10880=CARTESIAN_POINT ( 'NONE',  ( -14.50000000000000000, -21.00000000000000355, 1.000000000000000000 ) ) ;
#10917=EDGE_CURVE ( 'NONE', #7723, #10445, #18903, .T. ) ;
#10929=ORIENTED_EDGE ( 'NONE', *, *, #16926, .T. ) ;
#10954=ORIENTED_EDGE ( 'NONE', *, *, #14474, .T. ) ;
#10962=LINE ( 'NONE', #17330, #12650 ) ;
#10964=CARTESIAN_POINT ( 'NONE',  ( 9.000000000000000000, -9.999999999999991118, 2.500000000000000000 ) ) ;
#10978=CARTESIAN_POINT ( 'NONE',  ( -11.99999999999999467, -17.50000000000000000, 4.000000000000000000 ) ) ;
#10985=DIRECTION ( 'NONE',  ( -0.000000000000000000, -0.000000000000000000, -1.000000000000000000 ) ) ;
#11012=PLANE ( 'NONE',  #1245 ) ;
#11020=CARTESIAN_POINT ( 'NONE',  ( 32.65117217603048516, 6.460468870412194420, 1.000000000000000000 ) ) ;
#11030=ORIENTED_EDGE ( 'NONE', *, *, #6322, .F. ) ;
#11040=AXIS2_PLACEMENT_3D ( 'NONE', #17131, #2810, #15560 ) ;
#11044=CARTESIAN_POINT ( 'NONE',  ( -14.99999999999999645, -30.00000000000000711, 1.000000000000000000 ) ) ;
#11061=VERTEX_POINT ( 'NONE', #4994 ) ;
#11078=ORIENTED_EDGE ( 'NONE', *, *, #9821, .F. ) ;
#11084=DIRECTION ( 'NONE',  ( 1.000000000000000000, 3.469446951953611033E-15, -0.000000000000000000 ) ) ;
#11096=LINE ( 'NONE', #15889, #10157 ) ;
#11122=DIRECTION ( 'NONE',  ( 0.000000000000000000, -0.000000000000000000, 1.000000000000000000 ) ) ;
#11131=ORIENTED_EDGE ( 'NONE', *, *, #6418, .F. ) ;
#11135=VERTEX_POINT ( 'NONE', #16390 ) ;
#11161=CARTESIAN_POINT ( 'NONE',  ( -9.999999999999998224, -30.00000000000000355, 1.000000000000000000 ) ) ;
#11165=EDGE_CURVE ( 'NONE', #6152, #3941, #7191, .T. ) ;
#11170=LINE ( 'NONE', #19133, #6313 ) ;
#11209=ORIENTED_EDGE ( 'NONE', *, *, #7759, .T. ) ;
#11214=CARTESIAN_POINT ( 'NONE',  ( 15.00000000000001421, -17.49999999999999645, 4.000000000000000000 ) ) ;
#11220=CARTESIAN_POINT ( 'NONE',  ( -9.999999999999996447, -34.99999999999999289, 1.000000000000000000 ) ) ;
#11223=VERTEX_POINT ( 'NONE', #8760 ) ;
#11250=ORIENTED_EDGE ( 'NONE', *, *, #6418, .T. ) ;
#11282=DIRECTION ( 'NONE',  ( 0.000000000000000000, 0.000000000000000000, -1.000000000000000000 ) ) ;
#11283=ORIENTED_EDGE ( 'NONE', *, *, #5387, .T. ) ;
#11306=VECTOR ( 'NONE', #6473, 1000.000000000000000 ) ;
#11307=ORIENTED_EDGE ( 'NONE', *, *, #13064, .T. ) ;
#11309=PLANE ( 'NONE',  #13450 ) ;
#11320=DIRECTION ( 'NONE',  ( 0.000000000000000000, 0.000000000000000000, -1.000000000000000000 ) ) ;
#11342=CARTESIAN_POINT ( 'NONE',  ( -14.99999999999998224, -17.49999999999999645, 4.000000000000000000 ) ) ;
#11391=EDGE_CURVE ( 'NONE', #1866, #20635, #20488, .T. ) ;
#11403=PLANE ( 'NONE',  #9058 ) ;
#11408=ORIENTED_EDGE ( 'NONE', *, *, #3787, .T. ) ;
#11425=SURFACE_STYLE_USAGE ( .BOTH. , #5048 ) ;
#11426=CARTESIAN_POINT ( 'NONE',  ( 12.00000000000000178, -26.50000000000000355, 4.000000000000000000 ) ) ;
#11484=VECTOR ( 'NONE', #15315, 1000.000000000000000 ) ;
#11490=CARTESIAN_POINT ( 'NONE',  ( -14.49999999999999645, -22.99999999999998579, 4.000000000000000000 ) ) ;
#11520=DIRECTION ( 'NONE',  ( 1.000000000000000000, 0.000000000000000000, -0.000000000000000000 ) ) ;
#11527=CARTESIAN_POINT ( 'NONE',  ( 14.49999999999999822, -23.00000000000001421, 1.000000000000000000 ) ) ;
#11567=DIRECTION ( 'NONE',  ( -1.000000000000000000, -2.312964634635730039E-15, 0.000000000000000000 ) ) ;
#11572=EDGE_CURVE ( 'NONE', #18339, #20096, #17746, .T. ) ;
#11596=LINE ( 'NONE', #10455, #2121 ) ;
#11603=CARTESIAN_POINT ( 'NONE',  ( -14.49999999999999645, -21.00000000000000355, 4.000000000000000000 ) ) ;
#11613=PLANE ( 'NONE',  #5776 ) ;
#11616=PLANE ( 'NONE',  #2956 ) ;
#11630=ORIENTED_EDGE ( 'NONE', *, *, #18332, .F. ) ;
#11662=EDGE_CURVE ( 'NONE', #911, #18185, #5597, .T. ) ;
#11664=CARTESIAN_POINT ( 'NONE',  ( -11.99999999999999822, -18.50000000000000355, 4.000000000000000000 ) ) ;
#11667=DIRECTION ( 'NONE',  ( -1.000000000000000000, -0.000000000000000000, -0.000000000000000000 ) ) ;
#11670=DIRECTION ( 'NONE',  ( 1.000000000000000000, 6.938893903907222067E-15, 0.000000000000000000 ) ) ;
#11672=AXIS2_PLACEMENT_3D ( 'NONE', #15891, #7945, #6391 ) ;
#11687=ADVANCED_FACE ( 'NONE', ( #11967 ), #8632, .T. ) ;
#11695=DIRECTION ( 'NONE',  ( 0.000000000000000000, 1.000000000000000000, 0.000000000000000000 ) ) ;
#11719=DIRECTION ( 'NONE',  ( 3.469446951953611033E-15, -1.000000000000000000, 0.000000000000000000 ) ) ;
#11723=VECTOR ( 'NONE', #7883, 1000.000000000000000 ) ;
#11733=LINE ( 'NONE', #3575, #6062 ) ;
#11747=DIRECTION ( 'NONE',  ( -0.000000000000000000, 1.000000000000000000, 0.000000000000000000 ) ) ;
#11749=VECTOR ( 'NONE', #12226, 1000.000000000000000 ) ;
#11754=EDGE_CURVE ( 'NONE', #8919, #4928, #4028, .T. ) ;
#11774=CARTESIAN_POINT ( 'NONE',  ( -15.49999999999999822, -20.99999999999999645, 4.000000000000000000 ) ) ;
#11781=LINE ( 'NONE', #6873, #17979 ) ;
#11798=ORIENTED_EDGE ( 'NONE', *, *, #7276, .F. ) ;
#11803=PLANE ( 'NONE',  #6465 ) ;
#11811=VERTEX_POINT ( 'NONE', #13537 ) ;
#11821=EDGE_LOOP ( 'NONE', ( #2150, #3611, #11078, #20124, #6258, #14614 ) ) ;
#11840=ORIENTED_EDGE ( 'NONE', *, *, #18715, .F. ) ;
#11843=CARTESIAN_POINT ( 'NONE',  ( 27.00000000000000000, 0.000000000000000000, 1.000000000000000000 ) ) ;
#11849=CARTESIAN_POINT ( 'NONE',  ( 5.000000000000000000, -12.50000000000000000, 4.500000000000000888 ) ) ;
#11871=PLANE ( 'NONE',  #4424 ) ;
#11872=ORIENTED_EDGE ( 'NONE', *, *, #19336, .F. ) ;
#11873=DIRECTION ( 'NONE',  ( -0.000000000000000000, -0.000000000000000000, -1.000000000000000000 ) ) ;
#11874=EDGE_LOOP ( 'NONE', ( #10954, #5447 ) ) ;
#11896=VERTEX_POINT ( 'NONE', #2974 ) ;
#11901=DIRECTION ( 'NONE',  ( 1.000000000000000000, 6.938893903907232322E-16, -0.000000000000000000 ) ) ;
#11911=FACE_OUTER_BOUND ( 'NONE', #9627, .T. ) ;
#11918=LINE ( 'NONE', #6812, #3421 ) ;
#11920=ORIENTED_EDGE ( 'NONE', *, *, #14564, .T. ) ;
#11927=FACE_OUTER_BOUND ( 'NONE', #17563, .T. ) ;
#11929=DIRECTION ( 'NONE',  ( -0.000000000000000000, -0.000000000000000000, -1.000000000000000000 ) ) ;
#11943=ORIENTED_EDGE ( 'NONE', *, *, #7312, .F. ) ;
#11949=CARTESIAN_POINT ( 'NONE',  ( -5.000000000000000000, -12.50000000000000000, 4.500000000000000888 ) ) ;
#11967=FACE_OUTER_BOUND ( 'NONE', #15788, .T. ) ;
#11977=CARTESIAN_POINT ( 'NONE',  ( 5.000000000000000000, -7.500000000000000000, 1.000000000000000000 ) ) ;
#12004=ORIENTED_EDGE ( 'NONE', *, *, #12469, .T. ) ;
#12005=CARTESIAN_POINT ( 'NONE',  ( 10.00000000000000533, -30.00000000000000355, 1.000000000000000000 ) ) ;
#12009=DIRECTION ( 'NONE',  ( -3.469446951953611033E-15, 1.000000000000000000, 0.000000000000000000 ) ) ;
#12010=CARTESIAN_POINT ( 'NONE',  ( -15.49999999999999822, -20.99999999999999645, 1.000000000000000000 ) ) ;
#12047=VERTEX_POINT ( 'NONE', #13763 ) ;
#12055=AXIS2_PLACEMENT_3D ( 'NONE', #16463, #8311, #16658 ) ;
#12114=VECTOR ( 'NONE', #3779, 1000.000000000000000 ) ;
#12147=FACE_OUTER_BOUND ( 'NONE', #16304, .T. ) ;
#12151=ORIENTED_EDGE ( 'NONE', *, *, #10426, .T. ) ;
#12173=DIRECTION ( 'NONE',  ( -0.000000000000000000, -0.000000000000000000, -1.000000000000000000 ) ) ;
#12190=CARTESIAN_POINT ( 'NONE',  ( 9.000000000000000000, -9.999999999999991118, 1.000000000000000000 ) ) ;
#12204=EDGE_LOOP ( 'NONE', ( #17950, #9923, #1893, #5498 ) ) ;
#12218=CARTESIAN_POINT ( 'NONE',  ( 0.000000000000000000, 0.000000000000000000, 4.000000000000000000 ) ) ;
#12219=CARTESIAN_POINT ( 'NONE',  ( -14.49999999999998579, -18.49999999999999645, 1.000000000000000000 ) ) ;
#12226=DIRECTION ( 'NONE',  ( 0.000000000000000000, 0.000000000000000000, 1.000000000000000000 ) ) ;
#12236=VERTEX_POINT ( 'NONE', #7809 ) ;
#12259=FACE_OUTER_BOUND ( 'NONE', #6991, .T. ) ;
#12275=EDGE_LOOP ( 'NONE', ( #16295, #4032, #1482, #11408 ) ) ;
#12291=CARTESIAN_POINT ( 'NONE',  ( -9.999999999999998224, -30.00000000000000355, 1.000000000000000000 ) ) ;
#12294=CARTESIAN_POINT ( 'NONE',  ( 5.000000000000000000, 0.000000000000000000, 0.000000000000000000 ) ) ;
#12305=ORIENTED_EDGE ( 'NONE', *, *, #6337, .T. ) ;
#12316=DIRECTION ( 'NONE',  ( 4.625929269271477434E-15, 1.000000000000000000, 0.000000000000000000 ) ) ;
#12322=ADVANCED_FACE ( 'NONE', ( #12147 ), #4100, .F. ) ;
#12364=DIRECTION ( 'NONE',  ( 1.000000000000000000, 6.938893903907232322E-16, -0.000000000000000000 ) ) ;
#12366=AXIS2_PLACEMENT_3D ( 'NONE', #4147, #6032, #18585 ) ;
#12374=PRODUCT_DEFINITION_FORMATION_WITH_SPECIFIED_SOURCE ( 'ANY', '', #2828, .NOT_KNOWN. ) ;
#12414=VECTOR ( 'NONE', #12839, 1000.000000000000000 ) ;
#12433=CARTESIAN_POINT ( 'NONE',  ( -12.00000000000000000, -25.49999999999998934, 1.000000000000000000 ) ) ;
#12437=PLANE ( 'NONE',  #16003 ) ;
#12439=VERTEX_POINT ( 'NONE', #13913 ) ;
#12441=DIRECTION ( 'NONE',  ( -1.000000000000000000, -2.312964634635730039E-15, 0.000000000000000000 ) ) ;
#12462=ORIENTED_EDGE ( 'NONE', *, *, #7451, .F. ) ;
#12467=CARTESIAN_POINT ( 'NONE',  ( 5.000000000000000000, -12.50000000000000000, 1.000000000000000000 ) ) ;
#12469=EDGE_CURVE ( 'NONE', #12236, #17290, #16004, .T. ) ;
#12501=FACE_OUTER_BOUND ( 'NONE', #19270, .T. ) ;
#12504=LINE ( 'NONE', #7401, #7030 ) ;
#12559=ORIENTED_EDGE ( 'NONE', *, *, #2467, .T. ) ;
#12564=DIRECTION ( 'NONE',  ( -1.000000000000000000, 4.625929269271477434E-15, 0.000000000000000000 ) ) ;
#12571=CARTESIAN_POINT ( 'NONE',  ( -9.999999999999996447, -34.99999999999999289, 0.000000000000000000 ) ) ;
#12616=ORIENTED_EDGE ( 'NONE', *, *, #3188, .T. ) ;
#12619=CARTESIAN_POINT ( 'NONE',  ( -4.000000000000000000, -8.500000000000000000, 1.000000000000000000 ) ) ;
#12650=VECTOR ( 'NONE', #17440, 1000.000000000000227 ) ;
#12654=DIRECTION ( 'NONE',  ( -0.000000000000000000, -0.000000000000000000, -1.000000000000000000 ) ) ;
#12692=ORIENTED_EDGE ( 'NONE', *, *, #11662, .F. ) ;
#12703=DIRECTION ( 'NONE',  ( 3.469446951953611033E-15, -1.000000000000000000, 0.000000000000000000 ) ) ;
#12719=ADVANCED_FACE ( 'NONE', ( #7010 ), #18203, .F. ) ;
#12726=VERTEX_POINT ( 'NONE', #11603 ) ;
#12733=DIRECTION ( 'NONE',  ( 1.000000000000000000, -0.000000000000000000, -0.000000000000000000 ) ) ;
#12742=ADVANCED_FACE ( 'NONE', ( #3555 ), #11403, .T. ) ;
#12752=VECTOR ( 'NONE', #5130, 1000.000000000000000 ) ;
#12756=STYLED_ITEM ( 'NONE', ( #754 ), #17773 ) ;
#12761=CARTESIAN_POINT ( 'NONE',  ( -11.99999999999999467, -17.50000000000000000, 4.000000000000000000 ) ) ;
#12792=ORIENTED_EDGE ( 'NONE', *, *, #9517, .F. ) ;
#12826=FACE_OUTER_BOUND ( 'NONE', #17505, .T. ) ;
#12832=CARTESIAN_POINT ( 'NONE',  ( 15.50000000000002132, -26.49999999999999645, 4.000000000000000000 ) ) ;
#12839=DIRECTION ( 'NONE',  ( 3.469446951953619119E-16, -1.000000000000000000, 0.000000000000000000 ) ) ;
#12850=PLANE ( 'NONE',  #3118 ) ;
#12864=AXIS2_PLACEMENT_3D ( 'NONE', #16235, #1901, #11520 ) ;
#12915=ORIENTED_EDGE ( 'NONE', *, *, #15424, .T. ) ;
#12921=LINE ( 'NONE', #581, #14064 ) ;
#12925=VERTEX_POINT ( 'NONE', #8889 ) ;
#12927=DIRECTION ( 'NONE',  ( 1.000000000000000000, 0.000000000000000000, 0.000000000000000000 ) ) ;
#12951=ORIENTED_EDGE ( 'NONE', *, *, #11165, .F. ) ;
#12965=FACE_OUTER_BOUND ( 'NONE', #12275, .T. ) ;
#12977=ORIENTED_EDGE ( 'NONE', *, *, #8729, .F. ) ;
#12989=FILL_AREA_STYLE_COLOUR ( '', #19466 ) ;
#12993=ORIENTED_EDGE ( 'NONE', *, *, #16161, .T. ) ;
#13010=DIRECTION ( 'NONE',  ( 4.625929269271477434E-15, 1.000000000000000000, 0.000000000000000000 ) ) ;
#13038=CARTESIAN_POINT ( 'NONE',  ( 5.000000000000000000, -7.500000000000000000, 1.000000000000000000 ) ) ;
#13052=VECTOR ( 'NONE', #16883, 1000.000000000000000 ) ;
#13059=EDGE_CURVE ( 'NONE', #7068, #1942, #17869, .T. ) ;
#13061=ORIENTED_EDGE ( 'NONE', *, *, #16926, .F. ) ;
#13064=EDGE_CURVE ( 'NONE', #2576, #7246, #14729, .T. ) ;
#13087=CARTESIAN_POINT ( 'NONE',  ( 4.000000000000000000, -8.500000000000000000, 1.000000000000000000 ) ) ;
#13108=ORIENTED_EDGE ( 'NONE', *, *, #8347, .T. ) ;
#13116=CARTESIAN_POINT ( 'NONE',  ( -9.000000000000000000, -9.999999999999992895, 1.000000000000000000 ) ) ;
#13129=VECTOR ( 'NONE', #4808, 1000.000000000000000 ) ;
#13140=ORIENTED_EDGE ( 'NONE', *, *, #1990, .T. ) ;
#13184=EDGE_LOOP ( 'NONE', ( #15243, #7511, #19793, #14908 ) ) ;
#13189=FACE_BOUND ( 'NONE', #2664, .T. ) ;
#13196=EDGE_CURVE ( 'NONE', #7246, #6003, #3599, .T. ) ;
#13205=ORIENTED_EDGE ( 'NONE', *, *, #13695, .F. ) ;
#13214=CARTESIAN_POINT ( 'NONE',  ( -14.49999999999999645, -21.00000000000000355, 4.000000000000000000 ) ) ;
#13228=VERTEX_POINT ( 'NONE', #19867 ) ;
#13241=CARTESIAN_POINT ( 'NONE',  ( 15.00000000000001599, -18.49999999999999645, 1.000000000000000000 ) ) ;
#13255=PRODUCT_CONTEXT ( 'NONE', #20183, 'mechanical' ) ;
#13278=VERTEX_POINT ( 'NONE', #18284 ) ;
#13283=EDGE_CURVE ( 'NONE', #4928, #19894, #8870, .T. ) ;
#13291=CARTESIAN_POINT ( 'NONE',  ( -4.000000000000000000, -12.50000000000000000, 1.000000000000000000 ) ) ;
#13319=CARTESIAN_POINT ( 'NONE',  ( 15.50000000000000178, -20.99999999999999645, 4.000000000000000000 ) ) ;
#13324=ORIENTED_EDGE ( 'NONE', *, *, #2999, .T. ) ;
#13328=AXIS2_PLACEMENT_3D ( 'NONE', #4696, #15676, #4281 ) ;
#13360=VERTEX_POINT ( 'NONE', #4259 ) ;
#13373=VECTOR ( 'NONE', #12654, 1000.000000000000000 ) ;
#13381=CARTESIAN_POINT ( 'NONE',  ( -14.99999999999998401, -25.49999999999999645, 1.000000000000000000 ) ) ;
#13391=LINE ( 'NONE', #14859, #1358 ) ;
#13412=FACE_OUTER_BOUND ( 'NONE', #6850, .T. ) ;
#13450=AXIS2_PLACEMENT_3D ( 'NONE', #16018, #3364, #20637 ) ;
#13461=ORIENTED_EDGE ( 'NONE', *, *, #10626, .T. ) ;
#13488=ORIENTED_EDGE ( 'NONE', *, *, #18048, .F. ) ;
#13496=CARTESIAN_POINT ( 'NONE',  ( 10.00000000000000355, -34.99999999999999289, 1.000000000000000000 ) ) ;
#13507=EDGE_CURVE ( 'NONE', #16884, #19883, #20688, .T. ) ;
#13537=CARTESIAN_POINT ( 'NONE',  ( -15.49999999999998046, -26.49999999999999645, 1.000000000000000000 ) ) ;
#13543=DIRECTION ( 'NONE',  ( 0.000000000000000000, 0.000000000000000000, 1.000000000000000000 ) ) ;
#13544=EDGE_LOOP ( 'NONE', ( #3894, #18805, #881, #17203 ) ) ;
#13548=CYLINDRICAL_SURFACE ( 'NONE', #4969, 59.99999999999998579 ) ;
#13561=DIRECTION ( 'NONE',  ( 5.204170427930446527E-15, -1.000000000000000000, 0.000000000000000000 ) ) ;
#13564=VERTEX_POINT ( 'NONE', #7818 ) ;
#13568=EDGE_CURVE ( 'NONE', #18720, #11223, #19016, .T. ) ;
#13580=CARTESIAN_POINT ( 'NONE',  ( -5.000000000000000000, -7.500000000000000000, 1.000000000000000000 ) ) ;
#13588=CARTESIAN_POINT ( 'NONE',  ( 9.000000000000000000, -9.999999999999991118, 2.500000000000000000 ) ) ;
#13611=DIRECTION ( 'NONE',  ( -3.469446951953611033E-15, 1.000000000000000000, 0.000000000000000000 ) ) ;
#13616=EDGE_CURVE ( 'NONE', #3941, #13949, #12921, .T. ) ;
#13641=ORIENTED_EDGE ( 'NONE', *, *, #7472, .T. ) ;
#13662=CARTESIAN_POINT ( 'NONE',  ( -14.49999999999998579, -18.49999999999999645, 4.000000000000000000 ) ) ;
#13695=EDGE_CURVE ( 'NONE', #1231, #1866, #4980, .T. ) ;
#13698=DIRECTION ( 'NONE',  ( -1.000000000000000000, 0.000000000000000000, 0.000000000000000000 ) ) ;
#13702=VECTOR ( 'NONE', #16329, 1000.000000000000000 ) ;
#13743=EDGE_CURVE ( 'NONE', #18598, #20560, #19433, .T. ) ;
#13763=CARTESIAN_POINT ( 'NONE',  ( -11.99999999999999822, -18.50000000000000355, 4.000000000000000000 ) ) ;
#13765=CARTESIAN_POINT ( 'NONE',  ( 15.50000000000000178, -23.00000000000000711, 4.000000000000000000 ) ) ;
#13801=CARTESIAN_POINT ( 'NONE',  ( 14.50000000000001243, -25.49999999999999645, 4.000000000000000000 ) ) ;
#13849=VERTEX_POINT ( 'NONE', #4234 ) ;
#13862=LINE ( 'NONE', #5724, #9288 ) ;
#13876=ORIENTED_EDGE ( 'NONE', *, *, #6264, .F. ) ;
#13885=DIRECTION ( 'NONE',  ( -1.000000000000000000, -2.312964634635731617E-15, 0.000000000000000000 ) ) ;
#13892=PLANE ( 'NONE',  #9745 ) ;
#13913=CARTESIAN_POINT ( 'NONE',  ( 11.99999999999999822, -17.50000000000000000, 4.000000000000000000 ) ) ;
#13915=VECTOR ( 'NONE', #12441, 1000.000000000000000 ) ;
#13918=ORIENTED_EDGE ( 'NONE', *, *, #18596, .T. ) ;
#13923=ADVANCED_FACE ( 'NONE', ( #9054 ), #11871, .T. ) ;
#13946=ORIENTED_EDGE ( 'NONE', *, *, #10196, .T. ) ;
#13949=VERTEX_POINT ( 'NONE', #2455 ) ;
#13952=EDGE_CURVE ( 'NONE', #2483, #13360, #4134, .T. ) ;
#13955=LINE ( 'NONE', #18790, #20567 ) ;
#13960=DIRECTION ( 'NONE',  ( 3.469446951953611033E-15, -1.000000000000000000, 0.000000000000000000 ) ) ;
#13995=AXIS2_PLACEMENT_3D ( 'NONE', #4351, #10736, #4554 ) ;
#13996=VECTOR ( 'NONE', #11667, 1000.000000000000000 ) ;
#14002=ORIENTED_EDGE ( 'NONE', *, *, #6868, .T. ) ;
#14011=LINE ( 'NONE', #9209, #15594 ) ;
#14056=CARTESIAN_POINT ( 'NONE',  ( -5.000000000000000000, -12.50000000000000000, 1.000000000000000000 ) ) ;
#14064=VECTOR ( 'NONE', #14496, 1000.000000000000000 ) ;
#14106=CARTESIAN_POINT ( 'NONE',  ( -14.99999999999999645, -30.00000000000000711, 1.000000000000000000 ) ) ;
#14111=EDGE_CURVE ( 'NONE', #1942, #7441, #17798, .T. ) ;
#14114=VERTEX_POINT ( 'NONE', #14056 ) ;
#14159=ORIENTED_EDGE ( 'NONE', *, *, #6972, .F. ) ;
#14176=ORIENTED_EDGE ( 'NONE', *, *, #4777, .F. ) ;
#14191=CARTESIAN_POINT ( 'NONE',  ( 14.50000000000000000, -20.99999999999998934, 4.000000000000000000 ) ) ;
#14193=CARTESIAN_POINT ( 'NONE',  ( -32.65117217603048516, 6.460468870412185538, 0.000000000000000000 ) ) ;
#14199=ORIENTED_EDGE ( 'NONE', *, *, #1110, .T. ) ;
#14202=ORIENTED_EDGE ( 'NONE', *, *, #17853, .F. ) ;
#14203=DIRECTION ( 'NONE',  ( 1.000000000000000000, 0.000000000000000000, 0.000000000000000000 ) ) ;
#14236=LINE ( 'NONE', #16031, #9401 ) ;
#14251=EDGE_CURVE ( 'NONE', #6572, #3927, #11918, .T. ) ;
#14280=ORIENTED_EDGE ( 'NONE', *, *, #4442, .T. ) ;
#14303=VECTOR ( 'NONE', #13010, 1000.000000000000000 ) ;
#14307=LINE ( 'NONE', #7844, #14471 ) ;
#14334=ORIENTED_EDGE ( 'NONE', *, *, #2999, .F. ) ;
#14336=VECTOR ( 'NONE', #15432, 1000.000000000000000 ) ;
#14343=VECTOR ( 'NONE', #15153, 1000.000000000000000 ) ;
#14414=VERTEX_POINT ( 'NONE', #4285 ) ;
#14423=PLANE ( 'NONE',  #9927 ) ;
#14424=DIRECTION ( 'NONE',  ( -0.000000000000000000, -0.000000000000000000, -1.000000000000000000 ) ) ;
#14450=LINE ( 'NONE', #4934, #10696 ) ;
#14471=VECTOR ( 'NONE', #10985, 1000.000000000000000 ) ;
#14474=EDGE_CURVE ( 'NONE', #2576, #8456, #5218, .T. ) ;
#14496=DIRECTION ( 'NONE',  ( 5.204170427930446527E-15, -1.000000000000000000, 0.000000000000000000 ) ) ;
#14506=CARTESIAN_POINT ( 'NONE',  ( -15.49999999999998046, -26.49999999999999645, 4.000000000000000000 ) ) ;
#14525=EDGE_CURVE ( 'NONE', #1942, #868, #4185, .T. ) ;
#14540=VECTOR ( 'NONE', #15482, 1000.000000000000000 ) ;
#14564=EDGE_CURVE ( 'NONE', #11135, #4871, #5864, .T. ) ;
#14578=FACE_OUTER_BOUND ( 'NONE', #19967, .T. ) ;
#14580=LINE ( 'NONE', #255, #6703 ) ;
#14601=LINE ( 'NONE', #13038, #13996 ) ;
#14614=ORIENTED_EDGE ( 'NONE', *, *, #254, .T. ) ;
#14644=EDGE_CURVE ( 'NONE', #13564, #911, #15272, .T. ) ;
#14651=CARTESIAN_POINT ( 'NONE',  ( -12.00000000000000000, -25.49999999999998934, 1.000000000000000000 ) ) ;
#14654=FACE_OUTER_BOUND ( 'NONE', #18697, .T. ) ;
#14683=DIRECTION ( 'NONE',  ( 1.000000000000000000, 6.938893903907232322E-16, 0.000000000000000000 ) ) ;
#14689=LINE ( 'NONE', #568, #9641 ) ;
#14704=DIRECTION ( 'NONE',  ( -1.000000000000000000, -2.312964634635756072E-15, 0.000000000000000000 ) ) ;
#14706=SHAPE_REPRESENTATION ( 'Cast Metal _ Plastic Body Housing', ( #18039 ), #14707 ) ;
#14707=( GEOMETRIC_REPRESENTATION_CONTEXT ( 3 ) GLOBAL_UNCERTAINTY_ASSIGNED_CONTEXT ( ( #18648 ) ) GLOBAL_UNIT_ASSIGNED_CONTEXT ( ( #2200, #7021, #2506 ) ) REPRESENTATION_CONTEXT ( 'NONE', 'WORKASPACE' ) );
#14729=LINE ( 'NONE', #3539, #17637 ) ;
#14748=DIRECTION ( 'NONE',  ( -6.938893903907222067E-15, 1.000000000000000000, 0.000000000000000000 ) ) ;
#14762=EDGE_CURVE ( 'NONE', #8919, #7660, #20516, .T. ) ;
#14807=ORIENTED_EDGE ( 'NONE', *, *, #18303, .T. ) ;
#14809=VERTEX_POINT ( 'NONE', #1978 ) ;
#14812=ORIENTED_EDGE ( 'NONE', *, *, #9606, .T. ) ;
#14817=FACE_OUTER_BOUND ( 'NONE', #6709, .T. ) ;
#14823=EDGE_LOOP ( 'NONE', ( #8610, #8132 ) ) ;
#14832=ORIENTED_EDGE ( 'NONE', *, *, #2467, .F. ) ;
#14834=ORIENTED_EDGE ( 'NONE', *, *, #6868, .F. ) ;
#14859=CARTESIAN_POINT ( 'NONE',  ( -14.49999999999999645, -21.00000000000000355, 4.000000000000000000 ) ) ;
#14865=VECTOR ( 'NONE', #2986, 1000.000000000000000 ) ;
#14903=VERTEX_POINT ( 'NONE', #722 ) ;
#14908=ORIENTED_EDGE ( 'NONE', *, *, #11754, .T. ) ;
#14911=PLANE ( 'NONE',  #6993 ) ;
#14924=EDGE_LOOP ( 'NONE', ( #11283, #9462, #5417, #6860 ) ) ;
#14930=ORIENTED_EDGE ( 'NONE', *, *, #6786, .F. ) ;
#14932=EDGE_CURVE ( 'NONE', #1434, #5711, #5629, .T. ) ;
#14937=VECTOR ( 'NONE', #16023, 1000.000000000000000 ) ;
#14948=ORIENTED_EDGE ( 'NONE', *, *, #11165, .T. ) ;
#14952=( LENGTH_UNIT ( ) NAMED_UNIT ( * ) SI_UNIT ( .MILLI., .METRE. ) );
#14967=VECTOR ( 'NONE', #8860, 1000.000000000000000 ) ;
#14981=CARTESIAN_POINT ( 'NONE',  ( -15.49999999999999822, -20.99999999999999645, 1.000000000000000000 ) ) ;
#14984=VECTOR ( 'NONE', #6847, 1000.000000000000000 ) ;
#14985=LINE ( 'NONE', #1924, #9316 ) ;
#15029=ORIENTED_EDGE ( 'NONE', *, *, #18172, .T. ) ;
#15066=VECTOR ( 'NONE', #15715, 1000.000000000000000 ) ;
#15114=ORIENTED_EDGE ( 'NONE', *, *, #7540, .T. ) ;
#15129=VECTOR ( 'NONE', #6076, 1000.000000000000000 ) ;
#15131=CARTESIAN_POINT ( 'NONE',  ( -14.99999999999999645, -30.00000000000000711, 0.000000000000000000 ) ) ;
#15140=DIRECTION ( 'NONE',  ( 1.000000000000000000, 0.000000000000000000, 0.000000000000000000 ) ) ;
#15150=LINE ( 'NONE', #2390, #668 ) ;
#15151=CARTESIAN_POINT ( 'NONE',  ( 15.50000000000000178, -23.00000000000000711, 4.000000000000000000 ) ) ;
#15153=DIRECTION ( 'NONE',  ( 1.000000000000000000, 0.000000000000000000, 0.000000000000000000 ) ) ;
#15159=LINE ( 'NONE', #13580, #11749 ) ;
#15164=ORIENTED_EDGE ( 'NONE', *, *, #5701, .F. ) ;
#15170=DIRECTION ( 'NONE',  ( 1.000000000000000000, 0.000000000000000000, 0.000000000000000000 ) ) ;
#15179=LINE ( 'NONE', #1244, #15968 ) ;
#15180=FACE_OUTER_BOUND ( 'NONE', #10723, .T. ) ;
#15193=FACE_OUTER_BOUND ( 'NONE', #12204, .T. ) ;
#15217=EDGE_LOOP ( 'NONE', ( #20693, #15309, #8149, #11209 ) ) ;
#15222=DIRECTION ( 'NONE',  ( -0.000000000000000000, -0.000000000000000000, -1.000000000000000000 ) ) ;
#15235=EDGE_CURVE ( 'NONE', #14114, #19732, #2359, .T. ) ;
#15240=CARTESIAN_POINT ( 'NONE',  ( 14.50000000000000000, -23.00000000000001421, 1.000000000000000000 ) ) ;
#15241=LINE ( 'NONE', #13662, #19040 ) ;
#15243=ORIENTED_EDGE ( 'NONE', *, *, #13283, .T. ) ;
#15251=CARTESIAN_POINT ( 'NONE',  ( 7.500000000000002665, -9.999999999999991118, 2.500000000000000000 ) ) ;
#15272=CIRCLE ( 'NONE', #17619, 59.99999999999998579 ) ;
#15275=DIRECTION ( 'NONE',  ( 0.000000000000000000, 0.000000000000000000, 1.000000000000000000 ) ) ;
#15291=CARTESIAN_POINT ( 'NONE',  ( 15.00000000000000355, -30.00000000000000000, 0.000000000000000000 ) ) ;
#15295=VECTOR ( 'NONE', #15329, 1000.000000000000000 ) ;
#15309=ORIENTED_EDGE ( 'NONE', *, *, #10313, .F. ) ;
#15315=DIRECTION ( 'NONE',  ( 1.000000000000000000, -2.312964634635752916E-15, 0.000000000000000000 ) ) ;
#15317=ORIENTED_EDGE ( 'NONE', *, *, #7719, .T. ) ;
#15329=DIRECTION ( 'NONE',  ( -0.000000000000000000, -0.000000000000000000, -1.000000000000000000 ) ) ;
#15353=LINE ( 'NONE', #20188, #8036 ) ;
#15380=CARTESIAN_POINT ( 'NONE',  ( -14.49999999999999645, -22.99999999999998579, 4.000000000000000000 ) ) ;
#15423=DIRECTION ( 'NONE',  ( -6.938893903907222067E-15, -1.000000000000000000, 0.000000000000000000 ) ) ;
#15424=EDGE_CURVE ( 'NONE', #4929, #13278, #13955, .T. ) ;
#15430=ORIENTED_EDGE ( 'NONE', *, *, #16707, .F. ) ;
#15432=DIRECTION ( 'NONE',  ( -0.000000000000000000, -0.000000000000000000, -1.000000000000000000 ) ) ;
#15433=MECHANICAL_DESIGN_GEOMETRIC_PRESENTATION_REPRESENTATION('',(#12756),#6917);
#15436=LINE ( 'NONE', #18582, #514 ) ;
#15459=CARTESIAN_POINT ( 'NONE',  ( 15.50000000000001776, -17.49999999999999645, 1.000000000000000000 ) ) ;
#15474=ORIENTED_EDGE ( 'NONE', *, *, #13743, .T. ) ;
#15482=DIRECTION ( 'NONE',  ( -0.000000000000000000, -0.000000000000000000, -1.000000000000000000 ) ) ;
#15518=VERTEX_POINT ( 'NONE', #5144 ) ;
#15526=EDGE_CURVE ( 'NONE', #10023, #14414, #9849, .T. ) ;
#15560=DIRECTION ( 'NONE',  ( -1.000000000000000000, 0.000000000000000000, -0.000000000000000000 ) ) ;
#15573=ORIENTED_EDGE ( 'NONE', *, *, #19975, .F. ) ;
#15575=CARTESIAN_POINT ( 'NONE',  ( -14.99999999999998401, -25.49999999999999645, 4.000000000000000000 ) ) ;
#15594=VECTOR ( 'NONE', #9006, 1000.000000000000000 ) ;
#15596=ORIENTED_EDGE ( 'NONE', *, *, #10058, .T. ) ;
#15599=ADVANCED_FACE ( 'NONE', ( #3471, #6723, #13189, #18992, #1516, #17414, #19585, #10063 ), #17302, .T. ) ;
#15608=DIRECTION ( 'NONE',  ( -0.000000000000000000, -0.000000000000000000, -1.000000000000000000 ) ) ;
#15646=ORIENTED_EDGE ( 'NONE', *, *, #10564, .F. ) ;
#15654=EDGE_CURVE ( 'NONE', #10445, #6014, #18893, .T. ) ;
#15676=DIRECTION ( 'NONE',  ( -1.000000000000000000, 3.469446951953619119E-16, 0.000000000000000000 ) ) ;
#15715=DIRECTION ( 'NONE',  ( 1.000000000000000000, 6.938893903907222067E-15, 0.000000000000000000 ) ) ;
#15786=VECTOR ( 'NONE', #4522, 1000.000000000000000 ) ;
#15788=EDGE_LOOP ( 'NONE', ( #11030, #15430, #11920, #8221 ) ) ;
#15798=ADVANCED_FACE ( 'NONE', ( #11927 ), #18321, .F. ) ;
#15812=CARTESIAN_POINT ( 'NONE',  ( -14.49999999999999645, -21.00000000000000355, 4.000000000000000000 ) ) ;
#15858=PLANE ( 'NONE',  #7091 ) ;
#15866=DIRECTION ( 'NONE',  ( -0.000000000000000000, -0.000000000000000000, -1.000000000000000000 ) ) ;
#15876=CARTESIAN_POINT ( 'NONE',  ( 10.00000000000000533, -30.00000000000000355, 0.000000000000000000 ) ) ;
#15889=CARTESIAN_POINT ( 'NONE',  ( -14.99999999999998046, -26.49999999999999645, 1.000000000000000000 ) ) ;
#15891=CARTESIAN_POINT ( 'NONE',  ( 15.50000000000000178, -20.99999999999999645, 4.000000000000000000 ) ) ;
#15905=PRODUCT_DEFINITION_CONTEXT ( 'detailed design', #6151, 'design' ) ;
#15909=FACE_OUTER_BOUND ( 'NONE', #5805, .T. ) ;
#15920=ORIENTED_EDGE ( 'NONE', *, *, #10110, .T. ) ;
#15921=AXIS2_PLACEMENT_3D ( 'NONE', #11849, #11747, #18140 ) ;
#15927=ORIENTED_EDGE ( 'NONE', *, *, #4442, .F. ) ;
#15930=CARTESIAN_POINT ( 'NONE',  ( -14.49999999999999645, -21.00000000000000355, 4.000000000000000000 ) ) ;
#15933=CARTESIAN_POINT ( 'NONE',  ( -7.500000000000000888, -9.999999999999992895, 2.500000000000000000 ) ) ;
#15935=AXIS2_PLACEMENT_3D ( 'NONE', #15812, #12564, #18964 ) ;
#15949=EDGE_CURVE ( 'NONE', #7068, #19990, #2617, .T. ) ;
#15968=VECTOR ( 'NONE', #18822, 1000.000000000000000 ) ;
#16003=AXIS2_PLACEMENT_3D ( 'NONE', #2923, #9301, #17350 ) ;
#16004=LINE ( 'NONE', #12761, #13373 ) ;
#16017=ORIENTED_EDGE ( 'NONE', *, *, #10426, .F. ) ;
#16018=CARTESIAN_POINT ( 'NONE',  ( 5.000000000000000000, -7.500000000000000000, 3.160254037844365094 ) ) ;
#16020=VECTOR ( 'NONE', #10842, 1000.000000000000000 ) ;
#16023=DIRECTION ( 'NONE',  ( -3.469446951953611033E-15, -1.000000000000000000, 0.000000000000000000 ) ) ;
#16031=CARTESIAN_POINT ( 'NONE',  ( -14.99999999999998579, -18.49999999999999645, 4.000000000000000000 ) ) ;
#16043=ADVANCED_FACE ( 'NONE', ( #1266 ), #17880, .F. ) ;
#16057=PLANE ( 'NONE',  #4193 ) ;
#16068=EDGE_CURVE ( 'NONE', #11811, #13228, #11096, .T. ) ;
#16076=CARTESIAN_POINT ( 'NONE',  ( 5.000000000000000000, -7.500000000000000000, 3.160254037844365094 ) ) ;
#16087=DIRECTION ( 'NONE',  ( -0.000000000000000000, -0.000000000000000000, -1.000000000000000000 ) ) ;
#16119=VECTOR ( 'NONE', #10180, 1000.000000000000000 ) ;
#16135=VECTOR ( 'NONE', #18313, 1000.000000000000000 ) ;
#16145=EDGE_CURVE ( 'NONE', #551, #14903, #8368, .T. ) ;
#16147=LINE ( 'NONE', #237, #11723 ) ;
#16156=CIRCLE ( 'NONE', #5115, 1.499999999999998668 ) ;
#16160=ORIENTED_EDGE ( 'NONE', *, *, #16689, .T. ) ;
#16161=EDGE_CURVE ( 'NONE', #16884, #20045, #5014, .T. ) ;
#16162=VECTOR ( 'NONE', #20464, 1000.000000000000000 ) ;
#16178=DIRECTION ( 'NONE',  ( -0.000000000000000000, -0.000000000000000000, -1.000000000000000000 ) ) ;
#16182=ORIENTED_EDGE ( 'NONE', *, *, #155, .T. ) ;
#16201=ORIENTED_EDGE ( 'NONE', *, *, #13952, .F. ) ;
#16229=DIRECTION ( 'NONE',  ( 0.000000000000000000, 0.000000000000000000, 1.000000000000000000 ) ) ;
#16235=CARTESIAN_POINT ( 'NONE',  ( 32.65117217603048516, 6.460468870412194420, 1.000000000000000000 ) ) ;
#16258=LINE ( 'NONE', #4011, #5989 ) ;
#16273=ORIENTED_EDGE ( 'NONE', *, *, #4754, .T. ) ;
#16275=DIRECTION ( 'NONE',  ( 1.000000000000000000, -0.000000000000000000, -0.000000000000000000 ) ) ;
#16286=EDGE_CURVE ( 'NONE', #17877, #12439, #11596, .T. ) ;
#16295=ORIENTED_EDGE ( 'NONE', *, *, #18172, .F. ) ;
#16299=ADVANCED_FACE ( 'NONE', ( #4068 ), #11803, .T. ) ;
#16304=EDGE_LOOP ( 'NONE', ( #10929, #10440, #6757, #2100 ) ) ;
#16320=EDGE_LOOP ( 'NONE', ( #18178, #16201, #16017, #890, #5140, #16709 ) ) ;
#16329=DIRECTION ( 'NONE',  ( 3.469446951953611033E-15, -1.000000000000000000, 0.000000000000000000 ) ) ;
#16331=CIRCLE ( 'NONE', #18005, 1.499999999999998668 ) ;
#16332=DIRECTION ( 'NONE',  ( -0.000000000000000000, -0.000000000000000000, -1.000000000000000000 ) ) ;
#16356=CARTESIAN_POINT ( 'NONE',  ( -14.99999999999999645, -30.00000000000000711, 0.000000000000000000 ) ) ;
#16360=PLANE ( 'NONE',  #12055 ) ;
#16390=CARTESIAN_POINT ( 'NONE',  ( 15.50000000000002132, -26.49999999999999645, 4.000000000000000000 ) ) ;
#16407=ORIENTED_EDGE ( 'NONE', *, *, #16659, .F. ) ;
#16463=CARTESIAN_POINT ( 'NONE',  ( 14.50000000000000000, -23.00000000000001421, 4.000000000000000000 ) ) ;
#16474=VERTEX_POINT ( 'NONE', #15459 ) ;
#16490=DIRECTION ( 'NONE',  ( 5.204170427930411817E-15, -1.000000000000000000, 0.000000000000000000 ) ) ;
#16498=ORIENTED_EDGE ( 'NONE', *, *, #8574, .T. ) ;
#16500=CARTESIAN_POINT ( 'NONE',  ( -14.49999999999999645, -22.99999999999998579, 1.000000000000000000 ) ) ;
#16523=ORIENTED_EDGE ( 'NONE', *, *, #13568, .T. ) ;
#16563=ORIENTED_EDGE ( 'NONE', *, *, #11662, .T. ) ;
#16578=DIRECTION ( 'NONE',  ( -1.000000000000000000, 0.000000000000000000, 0.000000000000000000 ) ) ;
#16583=DIRECTION ( 'NONE',  ( -1.000000000000000000, -2.312964634635731617E-15, 0.000000000000000000 ) ) ;
#16625=AXIS2_PLACEMENT_3D ( 'NONE', #16702, #7097, #15140 ) ;
#16633=CARTESIAN_POINT ( 'NONE',  ( 11.99999999999999822, -25.50000000000000355, 4.000000000000000000 ) ) ;
#16635=EDGE_CURVE ( 'NONE', #200, #17877, #4579, .T. ) ;
#16643=ADVANCED_FACE ( 'NONE', ( #1036 ), #5849, .F. ) ;
#16648=ORIENTED_EDGE ( 'NONE', *, *, #520, .T. ) ;
#16653=VECTOR ( 'NONE', #18400, 1000.000000000000000 ) ;
#16658=DIRECTION ( 'NONE',  ( -1.000000000000000000, -6.938893903907222067E-15, 0.000000000000000000 ) ) ;
#16659=EDGE_CURVE ( 'NONE', #4928, #3941, #7728, .T. ) ;
#16678=ORIENTED_EDGE ( 'NONE', *, *, #18688, .T. ) ;
#16689=EDGE_CURVE ( 'NONE', #12925, #551, #4885, .T. ) ;
#16702=CARTESIAN_POINT ( 'NONE',  ( 9.000000000000000000, -9.999999999999991118, 1.000000000000000000 ) ) ;
#16705=ORIENTED_EDGE ( 'NONE', *, *, #18860, .F. ) ;
#16707=EDGE_CURVE ( 'NONE', #11135, #13949, #9496, .T. ) ;
#16709=ORIENTED_EDGE ( 'NONE', *, *, #6786, .T. ) ;
#16718=AXIS2_PLACEMENT_3D ( 'NONE', #4201, #16853, #7242 ) ;
#16739=LINE ( 'NONE', #10474, #9046 ) ;
#16746=LINE ( 'NONE', #18635, #19090 ) ;
#16748=( NAMED_UNIT ( * ) PLANE_ANGLE_UNIT ( ) SI_UNIT ( $, .RADIAN. ) );
#16762=DIRECTION ( 'NONE',  ( 0.000000000000000000, 0.000000000000000000, 1.000000000000000000 ) ) ;
#16764=FACE_OUTER_BOUND ( 'NONE', #3465, .T. ) ;
#16791=ADVANCED_FACE ( 'NONE', ( #14817 ), #491, .T. ) ;
#16800=LINE ( 'NONE', #2469, #14967 ) ;
#16806=ORIENTED_EDGE ( 'NONE', *, *, #18048, .T. ) ;
#16814=SHAPE_DEFINITION_REPRESENTATION ( #2006, #14706 ) ;
#16815=ORIENTED_EDGE ( 'NONE', *, *, #3188, .F. ) ;
#16839=SURFACE_STYLE_USAGE ( .BOTH. , #18310 ) ;
#16840=ORIENTED_EDGE ( 'NONE', *, *, #10564, .T. ) ;
#16852=EDGE_CURVE ( 'NONE', #6003, #7246, #4189, .T. ) ;
#16853=DIRECTION ( 'NONE',  ( 1.000000000000000000, 5.204170427930411817E-15, -0.000000000000000000 ) ) ;
#16860=CARTESIAN_POINT ( 'NONE',  ( 15.00000000000001421, -25.49999999999999645, 4.000000000000000000 ) ) ;
#16867=DIRECTION ( 'NONE',  ( -1.000000000000000000, -2.312964634635730039E-15, 0.000000000000000000 ) ) ;
#16872=DIRECTION ( 'NONE',  ( -0.000000000000000000, -0.000000000000000000, -1.000000000000000000 ) ) ;
#16883=DIRECTION ( 'NONE',  ( -0.000000000000000000, -0.000000000000000000, -1.000000000000000000 ) ) ;
#16884=VERTEX_POINT ( 'NONE', #12291 ) ;
#16890=ADVANCED_FACE ( 'NONE', ( #9164 ), #20260, .F. ) ;
#16926=EDGE_CURVE ( 'NONE', #5036, #11811, #15436, .T. ) ;
#16937=CARTESIAN_POINT ( 'NONE',  ( 15.00000000000001776, -26.49999999999999645, 4.000000000000000000 ) ) ;
#16960=UNCERTAINTY_MEASURE_WITH_UNIT (LENGTH_MEASURE( 1.000000000000000082E-05 ), #14952, 'distance_accuracy_value', 'NONE');
#16963=DIRECTION ( 'NONE',  ( 0.000000000000000000, 1.000000000000000000, 0.000000000000000000 ) ) ;
#16964=ADVANCED_FACE ( 'NONE', ( #12501 ), #10625, .F. ) ;
#16982=ORIENTED_EDGE ( 'NONE', *, *, #18688, .F. ) ;
#16984=CARTESIAN_POINT ( 'NONE',  ( 15.00000000000001776, -26.49999999999999645, 4.000000000000000000 ) ) ;
#16986=ORIENTED_EDGE ( 'NONE', *, *, #19336, .T. ) ;
#17028=CARTESIAN_POINT ( 'NONE',  ( 14.50000000000001243, -18.49999999999999645, 1.000000000000000000 ) ) ;
#17041=DIRECTION ( 'NONE',  ( -3.469446951953611033E-15, 1.000000000000000000, 0.000000000000000000 ) ) ;
#17076=ADVANCED_FACE ( 'NONE', ( #14578 ), #9671, .T. ) ;
#17089=CARTESIAN_POINT ( 'NONE',  ( 11.99999999999999822, -25.50000000000000355, 1.000000000000000000 ) ) ;
#17096=EDGE_LOOP ( 'NONE', ( #16498, #4313, #1276, #14202, #16982, #16523 ) ) ;
#17100=DIRECTION ( 'NONE',  ( 1.000000000000000000, 0.000000000000000000, 0.000000000000000000 ) ) ;
#17110=CARTESIAN_POINT ( 'NONE',  ( -10.49999999999999822, -9.999999999999992895, 2.500000000000000000 ) ) ;
#17131=CARTESIAN_POINT ( 'NONE',  ( 0.000000000000000000, 0.000000000000000000, 4.000000000000000000 ) ) ;
#17149=ORIENTED_EDGE ( 'NONE', *, *, #10082, .F. ) ;
#17154=ADVANCED_FACE ( 'NONE', ( #3399 ), #16057, .T. ) ;
#17163=CARTESIAN_POINT ( 'NONE',  ( -15.50000000000000000, -22.99999999999999289, 1.000000000000000000 ) ) ;
#17180=LINE ( 'NONE', #5793, #18084 ) ;
#17181=LINE ( 'NONE', #7669, #19906 ) ;
#17183=CARTESIAN_POINT ( 'NONE',  ( 15.50000000000000178, -20.99999999999999645, 1.000000000000000000 ) ) ;
#17200=ORIENTED_EDGE ( 'NONE', *, *, #16068, .T. ) ;
#17203=ORIENTED_EDGE ( 'NONE', *, *, #14111, .T. ) ;
#17206=PLANE ( 'NONE',  #13995 ) ;
#17223=DIRECTION ( 'NONE',  ( 3.469446951953619119E-16, -1.000000000000000000, 0.000000000000000000 ) ) ;
#17244=ORIENTED_EDGE ( 'NONE', *, *, #18303, .F. ) ;
#17290=VERTEX_POINT ( 'NONE', #2033 ) ;
#17302=PLANE ( 'NONE',  #12864 ) ;
#17327=AXIS2_PLACEMENT_3D ( 'NONE', #9901, #1953, #12927 ) ;
#17330=CARTESIAN_POINT ( 'NONE',  ( -4.000000000000000000, -8.500000000000000000, 2.392927049865408495 ) ) ;
#17338=CARTESIAN_POINT ( 'NONE',  ( 12.00000000000000178, -18.50000000000000355, 4.000000000000000000 ) ) ;
#17350=DIRECTION ( 'NONE',  ( -1.000000000000000000, -2.312964634635756072E-15, 0.000000000000000000 ) ) ;
#17355=CARTESIAN_POINT ( 'NONE',  ( 0.000000000000000000, 0.000000000000000000, 4.000000000000000000 ) ) ;
#17361=COLOUR_RGB ( '', 0.31764706, 0.68627451, 0.89019608) ;
#17374=VECTOR ( 'NONE', #12316, 1000.000000000000000 ) ;
#17389=DIRECTION ( 'NONE',  ( -1.000000000000000000, 0.000000000000000000, 0.000000000000000000 ) ) ;
#17393=ORIENTED_EDGE ( 'NONE', *, *, #4754, .F. ) ;
#17396=CARTESIAN_POINT ( 'NONE',  ( 15.50000000000000178, -23.00000000000000711, 1.000000000000000000 ) ) ;
#17414=FACE_BOUND ( 'NONE', #1408, .T. ) ;
#17440=DIRECTION ( 'NONE',  ( 0.000000000000000000, -0.9659258262890672020, 0.2588190451025245142 ) ) ;
#17461=VECTOR ( 'NONE', #533, 1000.000000000000000 ) ;
#17469=FACE_OUTER_BOUND ( 'NONE', #15217, .T. ) ;
#17473=VECTOR ( 'NONE', #11719, 1000.000000000000000 ) ;
#17492=FACE_OUTER_BOUND ( 'NONE', #1869, .T. ) ;
#17505=EDGE_LOOP ( 'NONE', ( #18357, #17393, #11630, #3007 ) ) ;
#17535=ADVANCED_BREP_SHAPE_REPRESENTATION ( '', ( #17773, #18039 ), #14707 ) ;
#17563=EDGE_LOOP ( 'NONE', ( #3505, #18108, #2378, #16563 ) ) ;
#17590=DIRECTION ( 'NONE',  ( -0.000000000000000000, -0.000000000000000000, -1.000000000000000000 ) ) ;
#17596=DIRECTION ( 'NONE',  ( 0.000000000000000000, 1.000000000000000000, 0.000000000000000000 ) ) ;
#17619=AXIS2_PLACEMENT_3D ( 'NONE', #19249, #4698, #14203 ) ;
#17637=VECTOR ( 'NONE', #19759, 1000.000000000000000 ) ;
#17641=DIRECTION ( 'NONE',  ( 1.000000000000000000, -0.000000000000000000, -0.000000000000000000 ) ) ;
#17658=ORIENTED_EDGE ( 'NONE', *, *, #6674, .F. ) ;
#17665=DIRECTION ( 'NONE',  ( -1.000000000000000000, 0.000000000000000000, -0.000000000000000000 ) ) ;
#17669=FACE_OUTER_BOUND ( 'NONE', #817, .T. ) ;
#17675=VECTOR ( 'NONE', #11670, 1000.000000000000000 ) ;
#17697=CIRCLE ( 'NONE', #990, 59.99999999999998579 ) ;
#17746=LINE ( 'NONE', #3412, #7720 ) ;
#17773=MANIFOLD_SOLID_BREP ( 'Cut-Extrude1', #4957 ) ;
#17775=ORIENTED_EDGE ( 'NONE', *, *, #15526, .T. ) ;
#17798=LINE ( 'NONE', #18674, #16162 ) ;
#17811=DIRECTION ( 'NONE',  ( -0.000000000000000000, -0.000000000000000000, -1.000000000000000000 ) ) ;
#17853=EDGE_CURVE ( 'NONE', #17894, #200, #20002, .T. ) ;
#17856=DIRECTION ( 'NONE',  ( 4.625929269271486900E-15, 1.000000000000000000, 0.000000000000000000 ) ) ;
#17869=LINE ( 'NONE', #11490, #6946 ) ;
#17877=VERTEX_POINT ( 'NONE', #17338 ) ;
#17880=PLANE ( 'NONE',  #19847 ) ;
#17894=VERTEX_POINT ( 'NONE', #3020 ) ;
#17904=CARTESIAN_POINT ( 'NONE',  ( -14.99999999999998224, -17.49999999999999645, 4.000000000000000000 ) ) ;
#17925=EDGE_CURVE ( 'NONE', #1866, #382, #15179, .T. ) ;
#17950=ORIENTED_EDGE ( 'NONE', *, *, #15654, .T. ) ;
#17952=DIRECTION ( 'NONE',  ( 0.000000000000000000, -1.000000000000000000, 0.000000000000000000 ) ) ;
#17953=CYLINDRICAL_SURFACE ( 'NONE', #4299, 1.499999999999996891 ) ;
#17965=VERTEX_POINT ( 'NONE', #14506 ) ;
#17969=EDGE_LOOP ( 'NONE', ( #5906, #5059, #9941, #14280 ) ) ;
#17972=ORIENTED_EDGE ( 'NONE', *, *, #10110, .F. ) ;
#17979=VECTOR ( 'NONE', #16490, 1000.000000000000000 ) ;
#17981=VECTOR ( 'NONE', #12733, 1000.000000000000000 ) ;
#17994=EDGE_LOOP ( 'NONE', ( #3923, #787, #7492, #12305 ) ) ;
#18002=DIRECTION ( 'NONE',  ( 1.000000000000000000, 5.204170427930446527E-15, -0.000000000000000000 ) ) ;
#18005=AXIS2_PLACEMENT_3D ( 'NONE', #13116, #19514, #5165 ) ;
#18039=AXIS2_PLACEMENT_3D ( 'NONE', #1793, #16229, #8180 ) ;
#18048=EDGE_CURVE ( 'NONE', #6863, #7723, #4788, .T. ) ;
#18084=VECTOR ( 'NONE', #16867, 1000.000000000000000 ) ;
#18086=VECTOR ( 'NONE', #1846, 1000.000000000000227 ) ;
#18090=EDGE_CURVE ( 'NONE', #9890, #17965, #11781, .T. ) ;
#18095=DIRECTION ( 'NONE',  ( 1.000000000000000000, 5.204170427930446527E-15, -0.000000000000000000 ) ) ;
#18108=ORIENTED_EDGE ( 'NONE', *, *, #16161, .F. ) ;
#18115=LINE ( 'NONE', #13087, #17461 ) ;
#18120=DIRECTION ( 'NONE',  ( -1.000000000000000000, -6.938893903907232322E-16, 0.000000000000000000 ) ) ;
#18140=DIRECTION ( 'NONE',  ( 0.000000000000000000, -0.000000000000000000, 1.000000000000000000 ) ) ;
#18145=FACE_OUTER_BOUND ( 'NONE', #599, .T. ) ;
#18165=FACE_OUTER_BOUND ( 'NONE', #688, .T. ) ;
#18172=EDGE_CURVE ( 'NONE', #2500, #19250, #902, .T. ) ;
#18178=ORIENTED_EDGE ( 'NONE', *, *, #8620, .T. ) ;
#18181=ORIENTED_EDGE ( 'NONE', *, *, #16659, .T. ) ;
#18185=VERTEX_POINT ( 'NONE', #15131 ) ;
#18193=DIRECTION ( 'NONE',  ( -5.204170427930446527E-15, 1.000000000000000000, 0.000000000000000000 ) ) ;
#18202=ORIENTED_EDGE ( 'NONE', *, *, #7276, .T. ) ;
#18203=PLANE ( 'NONE',  #10055 ) ;
#18212=ORIENTED_EDGE ( 'NONE', *, *, #13507, .F. ) ;
#18217=EDGE_CURVE ( 'NONE', #20635, #14903, #16800, .T. ) ;
#18234=DIRECTION ( 'NONE',  ( 2.312964634635730039E-15, -1.000000000000000000, 0.000000000000000000 ) ) ;
#18246=LINE ( 'NONE', #13214, #10401 ) ;
#18262=CARTESIAN_POINT ( 'NONE',  ( 15.50000000000000178, -20.99999999999999645, 4.000000000000000000 ) ) ;
#18271=AXIS2_PLACEMENT_3D ( 'NONE', #12190, #2566, #9263 ) ;
#18284=CARTESIAN_POINT ( 'NONE',  ( -4.000000000000000000, -8.500000000000000000, 1.000000000000000000 ) ) ;
#18292=DIRECTION ( 'NONE',  ( 1.000000000000000000, 0.000000000000000000, -0.000000000000000000 ) ) ;
#18299=ORIENTED_EDGE ( 'NONE', *, *, #7387, .F. ) ;
#18303=EDGE_CURVE ( 'NONE', #17894, #2477, #4356, .T. ) ;
#18305=CARTESIAN_POINT ( 'NONE',  ( 10.00000000000000355, -34.99999999999999289, 1.000000000000000000 ) ) ;
#18309=DIRECTION ( 'NONE',  ( -0.000000000000000000, -0.000000000000000000, -1.000000000000000000 ) ) ;
#18310=SURFACE_SIDE_STYLE ('',( #5654 ) ) ;
#18313=DIRECTION ( 'NONE',  ( 5.204170427930446527E-15, -1.000000000000000000, 0.000000000000000000 ) ) ;
#18316=DIRECTION ( 'NONE',  ( -0.000000000000000000, -0.000000000000000000, -1.000000000000000000 ) ) ;
#18321=PLANE ( 'NONE',  #5183 ) ;
#18331=VECTOR ( 'NONE', #16087, 1000.000000000000000 ) ;
#18332=EDGE_CURVE ( 'NONE', #14809, #382, #13862, .T. ) ;
#18339=VERTEX_POINT ( 'NONE', #17110 ) ;
#18346=DIRECTION ( 'NONE',  ( -0.000000000000000000, -0.000000000000000000, -1.000000000000000000 ) ) ;
#18357=ORIENTED_EDGE ( 'NONE', *, *, #15235, .F. ) ;
#18400=DIRECTION ( 'NONE',  ( -0.000000000000000000, -0.000000000000000000, -1.000000000000000000 ) ) ;
#18412=ORIENTED_EDGE ( 'NONE', *, *, #10626, .F. ) ;
#18452=VECTOR ( 'NONE', #253, 1000.000000000000000 ) ;
#18509=DIRECTION ( 'NONE',  ( 0.000000000000000000, 0.000000000000000000, 1.000000000000000000 ) ) ;
#18544=CARTESIAN_POINT ( 'NONE',  ( 12.00000000000000178, -26.50000000000000355, 4.000000000000000000 ) ) ;
#18547=DIRECTION ( 'NONE',  ( 1.000000000000000000, -3.469446951953611033E-15, 0.000000000000000000 ) ) ;
#18550=CYLINDRICAL_SURFACE ( 'NONE', #19349, 1.499999999999999556 ) ;
#18582=CARTESIAN_POINT ( 'NONE',  ( -15.49999999999999822, -22.99999999999999289, 1.000000000000000000 ) ) ;
#18585=DIRECTION ( 'NONE',  ( -1.000000000000000000, 0.000000000000000000, 0.000000000000000000 ) ) ;
#18596=EDGE_CURVE ( 'NONE', #1231, #14809, #19209, .T. ) ;
#18598=VERTEX_POINT ( 'NONE', #6229 ) ;
#18607=EDGE_CURVE ( 'NONE', #19894, #3922, #9881, .T. ) ;
#18608=CARTESIAN_POINT ( 'NONE',  ( 14.50000000000000000, -20.99999999999998934, 1.000000000000000000 ) ) ;
#18609=AXIS2_PLACEMENT_3D ( 'NONE', #872, #2228, #10181 ) ;
#18635=CARTESIAN_POINT ( 'NONE',  ( -27.00000000000000000, 0.000000000000000000, 1.000000000000000000 ) ) ;
#18648=UNCERTAINTY_MEASURE_WITH_UNIT (LENGTH_MEASURE( 1.000000000000000082E-05 ), #2200, 'distance_accuracy_value', 'NONE');
#18655=CARTESIAN_POINT ( 'NONE',  ( 10.00000000000000533, -30.00000000000000355, 1.000000000000000000 ) ) ;
#18659=CARTESIAN_POINT ( 'NONE',  ( -11.99999999999999645, -26.49999999999998934, 4.000000000000000000 ) ) ;
#18673=ORIENTED_EDGE ( 'NONE', *, *, #4875, .F. ) ;
#18674=CARTESIAN_POINT ( 'NONE',  ( -14.49999999999998401, -25.49999999999999645, 4.000000000000000000 ) ) ;
#18677=LINE ( 'NONE', #4345, #9106 ) ;
#18688=EDGE_CURVE ( 'NONE', #18720, #17894, #14689, .T. ) ;
#18690=CARTESIAN_POINT ( 'NONE',  ( 14.50000000000000000, -20.99999999999998934, 4.000000000000000000 ) ) ;
#18697=EDGE_LOOP ( 'NONE', ( #20606, #20589, #10104, #12915 ) ) ;
#18715=EDGE_CURVE ( 'NONE', #19461, #6659, #2235, .T. ) ;
#18720=VERTEX_POINT ( 'NONE', #13319 ) ;
#18790=CARTESIAN_POINT ( 'NONE',  ( -4.000000000000000000, -12.50000000000000000, 1.000000000000000000 ) ) ;
#18805=ORIENTED_EDGE ( 'NONE', *, *, #15949, .F. ) ;
#18822=DIRECTION ( 'NONE',  ( -1.000000000000000000, -0.000000000000000000, -0.000000000000000000 ) ) ;
#18831=PLANE ( 'NONE',  #13328 ) ;
#18858=CARTESIAN_POINT ( 'NONE',  ( 4.000000000000000000, -8.500000000000000000, 2.392927049865408495 ) ) ;
#18860=EDGE_CURVE ( 'NONE', #11896, #13228, #10600, .T. ) ;
#18861=ORIENTED_EDGE ( 'NONE', *, *, #6674, .T. ) ;
#18893=LINE ( 'NONE', #4552, #14865 ) ;
#18897=DIRECTION ( 'NONE',  ( 5.204170427930411817E-15, -1.000000000000000000, 0.000000000000000000 ) ) ;
#18901=FACE_OUTER_BOUND ( 'NONE', #9250, .T. ) ;
#18903=CIRCLE ( 'NONE', #9870, 59.99999999999998579 ) ;
#18919=CARTESIAN_POINT ( 'NONE',  ( -14.49999999999999645, -21.00000000000000355, 1.000000000000000000 ) ) ;
#18921=EDGE_CURVE ( 'NONE', #19883, #4642, #10819, .T. ) ;
#18962=FACE_OUTER_BOUND ( 'NONE', #198, .T. ) ;
#18964=DIRECTION ( 'NONE',  ( -4.625929269271477434E-15, -1.000000000000000000, 0.000000000000000000 ) ) ;
#18992=FACE_OUTER_BOUND ( 'NONE', #2832, .T. ) ;
#19001=CARTESIAN_POINT ( 'NONE',  ( 15.00000000000000000, 0.000000000000000000, 1.000000000000000000 ) ) ;
#19009=VECTOR ( 'NONE', #5077, 1000.000000000000000 ) ;
#19011=ORIENTED_EDGE ( 'NONE', *, *, #4317, .T. ) ;
#19013=DIRECTION ( 'NONE',  ( 0.000000000000000000, 0.000000000000000000, -1.000000000000000000 ) ) ;
#19016=LINE ( 'NONE', #3111, #5969 ) ;
#19024=VECTOR ( 'NONE', #1255, 1000.000000000000000 ) ;
#19028=DIRECTION ( 'NONE',  ( 4.625929269271486900E-15, 1.000000000000000000, 0.000000000000000000 ) ) ;
#19040=VECTOR ( 'NONE', #20072, 1000.000000000000000 ) ;
#19049=DIRECTION ( 'NONE',  ( 0.000000000000000000, 0.000000000000000000, 1.000000000000000000 ) ) ;
#19070=ADVANCED_FACE ( 'NONE', ( #535 ), #11616, .F. ) ;
#19090=VECTOR ( 'NONE', #11929, 1000.000000000000000 ) ;
#19109=CARTESIAN_POINT ( 'NONE',  ( -9.000000000000000000, -9.999999999999992895, 2.500000000000000000 ) ) ;
#19133=CARTESIAN_POINT ( 'NONE',  ( 15.50000000000001776, -17.49999999999999645, 4.000000000000000000 ) ) ;
#19138=DIRECTION ( 'NONE',  ( -1.000000000000000000, 0.000000000000000000, 0.000000000000000000 ) ) ;
#19158=CARTESIAN_POINT ( 'NONE',  ( 4.000000000000000000, -12.50000000000000000, 3.464723819589916154 ) ) ;
#19198=ORIENTED_EDGE ( 'NONE', *, *, #13059, .F. ) ;
#19209=LINE ( 'NONE', #20673, #628 ) ;
#19249=CARTESIAN_POINT ( 'NONE',  ( 32.65117217603048516, 6.460468870412194420, 1.000000000000000000 ) ) ;
#19250=VERTEX_POINT ( 'NONE', #2195 ) ;
#19270=EDGE_LOOP ( 'NONE', ( #10384, #8837, #17149, #3644 ) ) ;
#19278=VECTOR ( 'NONE', #5371, 1000.000000000000000 ) ;
#19309=VECTOR ( 'NONE', #19872, 1000.000000000000000 ) ;
#19313=DIRECTION ( 'NONE',  ( -1.000000000000000000, -0.000000000000000000, -0.000000000000000000 ) ) ;
#19325=DIRECTION ( 'NONE',  ( -2.312964634635756072E-15, 1.000000000000000000, 0.000000000000000000 ) ) ;
#19336=EDGE_CURVE ( 'NONE', #3190, #15518, #7016, .T. ) ;
#19348=ORIENTED_EDGE ( 'NONE', *, *, #7387, .T. ) ;
#19349=AXIS2_PLACEMENT_3D ( 'NONE', #4214, #18346, #4010 ) ;
#19351=VECTOR ( 'NONE', #16872, 1000.000000000000000 ) ;
#19368=DIRECTION ( 'NONE',  ( 2.312964634635731617E-15, -1.000000000000000000, 0.000000000000000000 ) ) ;
#19377=EDGE_LOOP ( 'NONE', ( #3972, #10358, #244, #2474 ) ) ;
#19378=EDGE_LOOP ( 'NONE', ( #17658, #4340, #16678, #14807 ) ) ;
#19390=SURFACE_STYLE_FILL_AREA ( #5461 ) ;
#19418=DIRECTION ( 'NONE',  ( -0.000000000000000000, -0.000000000000000000, -1.000000000000000000 ) ) ;
#19426=EDGE_CURVE ( 'NONE', #911, #16884, #10667, .T. ) ;
#19433=LINE ( 'NONE', #9895, #10421 ) ;
#19461=VERTEX_POINT ( 'NONE', #10880 ) ;
#19466=COLOUR_RGB ( '', 0.31764706, 0.68627451, 0.89019608) ;
#19475=CARTESIAN_POINT ( 'NONE',  ( 15.00000000000001599, -18.49999999999999645, 4.000000000000000000 ) ) ;
#19512=LINE ( 'NONE', #19820, #16119 ) ;
#19514=DIRECTION ( 'NONE',  ( 0.000000000000000000, 0.000000000000000000, 1.000000000000000000 ) ) ;
#19540=DIRECTION ( 'NONE',  ( -4.625929269271477434E-15, -1.000000000000000000, 0.000000000000000000 ) ) ;
#19562=ADVANCED_FACE ( 'NONE', ( #1460 ), #18831, .F. ) ;
#19565=AXIS2_PLACEMENT_3D ( 'NONE', #4144, #7497, #4556 ) ;
#19581=CARTESIAN_POINT ( 'NONE',  ( -14.99999999999998046, -26.49999999999999645, 4.000000000000000000 ) ) ;
#19585=FACE_BOUND ( 'NONE', #20441, .T. ) ;
#19588=ADVANCED_FACE ( 'NONE', ( #7839 ), #4394, .T. ) ;
#19595=EDGE_CURVE ( 'NONE', #12236, #12047, #2719, .T. ) ;
#19597=ADVANCED_FACE ( 'NONE', ( #6069 ), #12437, .T. ) ;
#19605=ORIENTED_EDGE ( 'NONE', *, *, #18332, .T. ) ;
#19636=CARTESIAN_POINT ( 'NONE',  ( -32.65117217603048516, 6.460468870412185538, 1.000000000000000000 ) ) ;
#19680=CARTESIAN_POINT ( 'NONE',  ( 4.000000000000000000, -8.500000000000000000, 2.392927049865408495 ) ) ;
#19684=AXIS2_PLACEMENT_3D ( 'NONE', #10964, #9394, #8033 ) ;
#19711=CARTESIAN_POINT ( 'NONE',  ( 14.50000000000001243, -25.49999999999999645, 4.000000000000000000 ) ) ;
#19732=VERTEX_POINT ( 'NONE', #8050 ) ;
#19759=DIRECTION ( 'NONE',  ( -0.000000000000000000, -0.000000000000000000, -1.000000000000000000 ) ) ;
#19793=ORIENTED_EDGE ( 'NONE', *, *, #14762, .F. ) ;
#19795=DIRECTION ( 'NONE',  ( -5.204170427930411817E-15, 1.000000000000000000, 0.000000000000000000 ) ) ;
#19820=CARTESIAN_POINT ( 'NONE',  ( 15.50000000000000178, -20.99999999999999645, 1.000000000000000000 ) ) ;
#19847=AXIS2_PLACEMENT_3D ( 'NONE', #3144, #6387, #1777 ) ;
#19867=CARTESIAN_POINT ( 'NONE',  ( -11.99999999999999645, -26.49999999999998934, 1.000000000000000000 ) ) ;
#19872=DIRECTION ( 'NONE',  ( 5.204170427930446527E-15, -1.000000000000000000, 0.000000000000000000 ) ) ;
#19883=VERTEX_POINT ( 'NONE', #8461 ) ;
#19892=VECTOR ( 'NONE', #16332, 1000.000000000000000 ) ;
#19894=VERTEX_POINT ( 'NONE', #19963 ) ;
#19906=VECTOR ( 'NONE', #10707, 1000.000000000000000 ) ;
#19963=CARTESIAN_POINT ( 'NONE',  ( 14.50000000000001243, -25.49999999999999645, 1.000000000000000000 ) ) ;
#19967=EDGE_LOOP ( 'NONE', ( #14930, #1820, #6357, #12004 ) ) ;
#19973=CARTESIAN_POINT ( 'NONE',  ( -4.000000000000000000, -8.500000000000000000, 1.000000000000000000 ) ) ;
#19975=EDGE_CURVE ( 'NONE', #11061, #2483, #15241, .T. ) ;
#19990=VERTEX_POINT ( 'NONE', #16500 ) ;
#19997=FACE_OUTER_BOUND ( 'NONE', #5627, .T. ) ;
#20000=LINE ( 'NONE', #5972, #1375 ) ;
#20002=LINE ( 'NONE', #14191, #6963 ) ;
#20004=PLANE ( 'NONE',  #10072 ) ;
#20019=ADVANCED_FACE ( 'NONE', ( #20563 ), #1607, .T. ) ;
#20043=CARTESIAN_POINT ( 'NONE',  ( -14.99999999999999645, -30.00000000000000711, 1.000000000000000000 ) ) ;
#20045=VERTEX_POINT ( 'NONE', #6317 ) ;
#20054=STYLED_ITEM ( 'NONE', ( #3874 ), #17535 ) ;
#20072=DIRECTION ( 'NONE',  ( -0.000000000000000000, -0.000000000000000000, -1.000000000000000000 ) ) ;
#20096=VERTEX_POINT ( 'NONE', #3183 ) ;
#20100=SHAPE_REPRESENTATION_RELATIONSHIP ( 'NONE' , 'NONE' ,  #14706, #17535 ) ;
#20124=ORIENTED_EDGE ( 'NONE', *, *, #155, .F. ) ;
#20135=DIRECTION ( 'NONE',  ( -0.000000000000000000, -0.000000000000000000, -1.000000000000000000 ) ) ;
#20147=DIRECTION ( 'NONE',  ( 2.312964634635730039E-15, -1.000000000000000000, 0.000000000000000000 ) ) ;
#20164=DIRECTION ( 'NONE',  ( 0.000000000000000000, -0.9659258262890672020, 0.2588190451025246253 ) ) ;
#20172=ORIENTED_EDGE ( 'NONE', *, *, #13616, .T. ) ;
#20183=APPLICATION_CONTEXT ( 'automotive_design' ) ;
#20188=CARTESIAN_POINT ( 'NONE',  ( 15.00000000000000355, -30.00000000000000000, 1.000000000000000000 ) ) ;
#20222=CARTESIAN_POINT ( 'NONE',  ( -32.65117217603048516, 6.460468870412185538, 1.000000000000000000 ) ) ;
#20245=ORIENTED_EDGE ( 'NONE', *, *, #6354, .T. ) ;
#20248=ORIENTED_EDGE ( 'NONE', *, *, #14644, .F. ) ;
#20249=EDGE_LOOP ( 'NONE', ( #11840, #7417, #19011, #16648 ) ) ;
#20260=PLANE ( 'NONE',  #5227 ) ;
#20262=LINE ( 'NONE', #5921, #5748 ) ;
#20274=ORIENTED_EDGE ( 'NONE', *, *, #15949, .T. ) ;
#20277=ORIENTED_EDGE ( 'NONE', *, *, #7472, .F. ) ;
#20327=PRODUCT_DEFINITION ( 'UNKNOWN', '', #12374, #15905 ) ;
#20352=ORIENTED_EDGE ( 'NONE', *, *, #14564, .F. ) ;
#20365=CIRCLE ( 'NONE', #17327, 1.499999999999998668 ) ;
#20379=VERTEX_POINT ( 'NONE', #11843 ) ;
#20386=VECTOR ( 'NONE', #13611, 1000.000000000000000 ) ;
#20411=DIRECTION ( 'NONE',  ( 1.000000000000000000, 0.000000000000000000, 0.000000000000000000 ) ) ;
#20430=EDGE_CURVE ( 'NONE', #4871, #4902, #8918, .T. ) ;
#20441=EDGE_LOOP ( 'NONE', ( #20245, #1604, #3236, #18181, #20172, #7414 ) ) ;
#20464=DIRECTION ( 'NONE',  ( -0.000000000000000000, -0.000000000000000000, -1.000000000000000000 ) ) ;
#20488=LINE ( 'NONE', #7712, #3307 ) ;
#20503=ADVANCED_FACE ( 'NONE', ( #13412 ), #5471, .F. ) ;
#20516=LINE ( 'NONE', #10134, #19309 ) ;
#20532=EDGE_CURVE ( 'NONE', #6863, #20379, #17697, .T. ) ;
#20560=VERTEX_POINT ( 'NONE', #18858 ) ;
#20563=FACE_OUTER_BOUND ( 'NONE', #20249, .T. ) ;
#20567=VECTOR ( 'NONE', #10841, 1000.000000000000000 ) ;
#20589=ORIENTED_EDGE ( 'NONE', *, *, #9355, .T. ) ;
#20600=DIRECTION ( 'NONE',  ( 0.000000000000000000, 0.000000000000000000, 1.000000000000000000 ) ) ;
#20604=LINE ( 'NONE', #9404, #12414 ) ;
#20606=ORIENTED_EDGE ( 'NONE', *, *, #10082, .T. ) ;
#20633=VECTOR ( 'NONE', #7867, 1000.000000000000000 ) ;
#20635=VERTEX_POINT ( 'NONE', #3776 ) ;
#20637=DIRECTION ( 'NONE',  ( 0.000000000000000000, 0.9659258262890672020, -0.2588190451025246808 ) ) ;
#20660=ORIENTED_EDGE ( 'NONE', *, *, #14932, .F. ) ;
#20673=CARTESIAN_POINT ( 'NONE',  ( 5.000000000000000000, -7.500000000000000000, 3.160254037844365094 ) ) ;
#20688=LINE ( 'NONE', #11161, #5636 ) ;
#20693=ORIENTED_EDGE ( 'NONE', *, *, #8729, .T. ) ;
ENDSEC;
END-ISO-10303-21;
